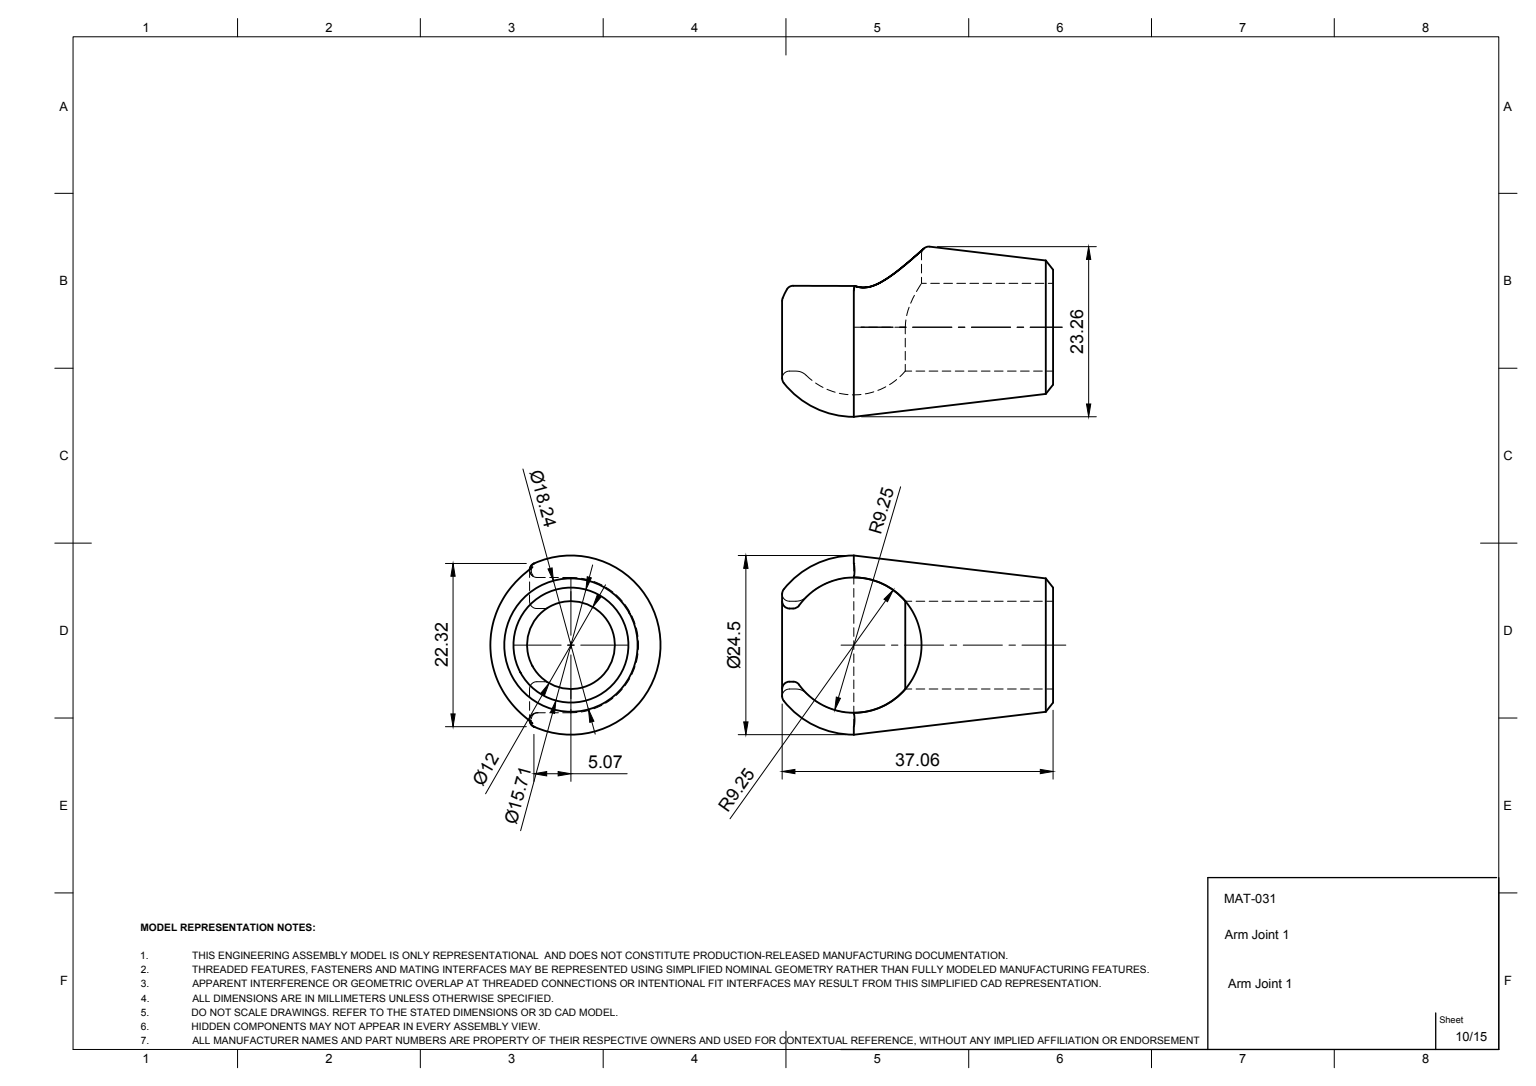
ISO-10303-21;
HEADER;
/* Generated by software containing ST-Developer
 * from STEP Tools, Inc. (www.steptools.com) 
 */

FILE_DESCRIPTION(
/* description */ ('STEP AP214'),
/* implementation_level */ '2;1');

FILE_NAME(
/* name */ 'Arm Joint 1.step',
/* time_stamp */ '2026-11-14T06:58:01-08:00',
/* author */ (''),
/* organization */ (''),
/* preprocessor_version */ 'ST-DEVELOPER v20.2',
/* originating_system */ 'Autodesk Translation Framework v15.17.0.0',
/* authorisation */ '');

FILE_SCHEMA (('AUTOMOTIVE_DESIGN { 1 0 10303 214 3 1 1 }'));
ENDSEC;

DATA;
#10=MECHANICAL_DESIGN_GEOMETRIC_PRESENTATION_REPRESENTATION('',(#1153),#38635);
#67=ELLIPSE('',#18082,0.093043907355238,0.0660721764139862);
#79=SPHERICAL_SURFACE('',#18062,1.);
#80=SPHERICAL_SURFACE('',#18074,9.25);
#81=SPHERICAL_SURFACE('',#18083,12.25);
#82=SPHERICAL_SURFACE('',#18107,1.);
#83=SPHERICAL_SURFACE('',#18111,1.);
#84=SPHERICAL_SURFACE('',#18115,1.);
#85=SPHERICAL_SURFACE('',#18118,1.);
#86=SPHERICAL_SURFACE('',#18123,1.);
#126=(
BOUNDED_SURFACE()
B_SPLINE_SURFACE(3,2,((#31255,#31256,#31257),(#31258,#31259,#31260),(#31261,
#31262,#31263),(#31264,#31265,#31266),(#31267,#31268,#31269),(#31270,#31271,
#31272),(#31273,#31274,#31275),(#31276,#31277,#31278),(#31279,#31280,#31281),
(#31282,#31283,#31284),(#31285,#31286,#31287),(#31288,#31289,#31290),(#31291,
#31292,#31293),(#31294,#31295,#31296),(#31297,#31298,#31299),(#31300,#31301,
#31302),(#31303,#31304,#31305),(#31306,#31307,#31308),(#31309,#31310,#31311),
(#31312,#31313,#31314),(#31315,#31316,#31317),(#31318,#31319,#31320),(#31321,
#31322,#31323),(#31324,#31325,#31326)),.UNSPECIFIED.,.F.,.F.,.F.)
B_SPLINE_SURFACE_WITH_KNOTS((4,2,2,2,2,2,2,2,2,2,2,4),(3,3),(-4.33680868994202E-19,
0.00199566610229966,0.00299349915344949,0.00399133220459933,0.00598699830689899,
0.00698483135804882,0.00748374788362374,0.00773320614641119,0.00785793527780492,
0.00792029984350179,0.00795148212635022,0.00798266440919865),(-8.88988013967173,
1.),.UNSPECIFIED.)
GEOMETRIC_REPRESENTATION_ITEM()
RATIONAL_B_SPLINE_SURFACE(((1.03673130903543,0.997934094247711,1.),(1.03429323702968,
0.998071220506301,1.),(1.03166096458261,0.99821926932168,1.),(1.02743039620336,
0.998457212258636,1.),(1.0259730109093,0.99853918104062,1.),(1.02296180766651,
0.998708542336582,1.),(1.02140250811888,0.998796243156116,1.),(1.01667872310722,
0.999061926435161,1.),(1.0134397522586,0.999244098230379,1.),(1.00845036900139,
0.999524719744889,1.),(1.00676184803489,0.99961968845875,1.),(1.00420736775411,
0.999763361952692,1.),(1.00335516609469,0.999811292950975,1.),(1.00207805691192,
0.999883122332401,1.),(1.00165222462761,0.999907072727549,1.),(1.00101619611475,
0.999942845342188,1.),(1.000804914933,0.999954728583493,1.),(1.00049166224454,
0.99997234708248,1.),(1.00038777606523,0.999978190028486,1.),(1.00023475952815,
0.999986796248967,1.),(1.00018401486096,0.999989650318224,1.),(1.00008917562832,
0.999994984430222,1.),(1.00003836348216,0.999997842294746,1.),(1.00003093298314,
0.999998260213712,1.)))
REPRESENTATION_ITEM('')
SURFACE()
);
#127=(
BOUNDED_SURFACE()
B_SPLINE_SURFACE(3,2,((#31328,#31329,#31330),(#31331,#31332,#31333),(#31334,
#31335,#31336),(#31337,#31338,#31339),(#31340,#31341,#31342),(#31343,#31344,
#31345),(#31346,#31347,#31348),(#31349,#31350,#31351),(#31352,#31353,#31354),
(#31355,#31356,#31357),(#31358,#31359,#31360),(#31361,#31362,#31363),(#31364,
#31365,#31366),(#31367,#31368,#31369),(#31370,#31371,#31372),(#31373,#31374,
#31375)),.UNSPECIFIED.,.F.,.F.,.F.)
B_SPLINE_SURFACE_WITH_KNOTS((4,2,2,2,2,2,2,4),(3,3),(-1.37073647788269E-16,
3.79857431933033E-5,7.59714863867437E-5,0.000151942972773624,0.000303885945547386,
0.000607771891094909,0.00121554378218996,0.00243108756438005),(-0.000101005518536674,
1.),.UNSPECIFIED.)
GEOMETRIC_REPRESENTATION_ITEM()
RATIONAL_B_SPLINE_SURFACE(((1.00000004220253,0.999791088022201,1.),(1.00000004430103,
0.999780699959677,1.),(1.00000006201562,0.999693008760642,1.),(1.00000010657676,
0.999472421084997,1.),(1.00000013303073,0.999341468019306,1.),(1.00000021861,
0.998917831394663,1.),(1.00000028470715,0.998590635693005,1.),(1.00000049900653,
0.997529805625635,1.),(1.00000066545063,0.996705869955465,1.),(1.00000123037801,
0.993909352546599,1.),(1.00000169504325,0.99160915523887,1.),(1.00000335151631,
0.983409241593269,1.),(1.00000480674396,0.976205537946754,1.),(1.00001025390194,
0.949240882635747,1.),(1.00001533088998,0.924108651696566,1.),(1.00002191434951,
0.891519048541741,1.)))
REPRESENTATION_ITEM('')
SURFACE()
);
#128=(
BOUNDED_SURFACE()
B_SPLINE_SURFACE(3,2,((#31377,#31378,#31379),(#31380,#31381,#31382),(#31383,
#31384,#31385),(#31386,#31387,#31388)),.UNSPECIFIED.,.F.,.F.,.F.)
B_SPLINE_SURFACE_WITH_KNOTS((4,4),(3,3),(-1.3918214625889E-5,0.00121512868205196),
(0.,1.00001391821463),.UNSPECIFIED.)
GEOMETRIC_REPRESENTATION_ITEM()
RATIONAL_B_SPLINE_SURFACE(((0.999999999999999,0.891779221283223,1.00000301248005),
(1.,0.884413245314419,1.00000321752252),(1.,0.87579683831728,1.00000345737252),
(1.,0.866200683852581,1.0000037244952)))
REPRESENTATION_ITEM('')
SURFACE()
);
#129=(
BOUNDED_SURFACE()
B_SPLINE_SURFACE(3,2,((#31400,#31401,#31402),(#31403,#31404,#31405),(#31406,
#31407,#31408),(#31409,#31410,#31411),(#31412,#31413,#31414),(#31415,#31416,
#31417),(#31418,#31419,#31420),(#31421,#31422,#31423),(#31424,#31425,#31426),
(#31427,#31428,#31429),(#31430,#31431,#31432),(#31433,#31434,#31435),(#31436,
#31437,#31438),(#31439,#31440,#31441)),.UNSPECIFIED.,.F.,.F.,.F.)
B_SPLINE_SURFACE_WITH_KNOTS((4,2,2,2,2,2,4),(3,3),(0.033103384374427,0.0355583288461946,
0.0367823574217915,0.0380063859973883,0.0392304145729851,0.0404544431485819,
0.0429025002997755),(0.,1.00000688732057),.UNSPECIFIED.)
GEOMETRIC_REPRESENTATION_ITEM()
RATIONAL_B_SPLINE_SURFACE(((1.,0.211850238456311,1.00001085648014),(1.,
0.211789774891773,1.000010857313),(1.,0.211720587176297,1.00001085826604),
(1.,0.21160403471626,1.0000108598715),(1.,0.211562868788471,1.00001086043855),
(1.,0.211477187752812,1.00001086161878),(1.,0.211433005503744,1.00001086222737),
(1.,0.211342033825223,1.00001086348047),(1.,0.211295244231205,1.00001086412498),
(1.,0.211199020809361,1.00001086545043),(1.,0.211149240972151,1.00001086613613),
(1.,0.21099910955097,1.00001086820413),(1.,0.210897693883658,1.0000108696011),
(1.,0.21079496787879,1.00001087101611)))
REPRESENTATION_ITEM('')
SURFACE()
);
#130=(
BOUNDED_SURFACE()
B_SPLINE_SURFACE(3,2,((#31518,#31519,#31520),(#31521,#31522,#31523),(#31524,
#31525,#31526),(#31527,#31528,#31529),(#31530,#31531,#31532),(#31533,#31534,
#31535),(#31536,#31537,#31538),(#31539,#31540,#31541),(#31542,#31543,#31544),
(#31545,#31546,#31547),(#31548,#31549,#31550),(#31551,#31552,#31553),(#31554,
#31555,#31556),(#31557,#31558,#31559),(#31560,#31561,#31562),(#31563,#31564,
#31565),(#31566,#31567,#31568),(#31569,#31570,#31571),(#31572,#31573,#31574),
(#31575,#31576,#31577),(#31578,#31579,#31580),(#31581,#31582,#31583),(#31584,
#31585,#31586),(#31587,#31588,#31589),(#31590,#31591,#31592),(#31593,#31594,
#31595),(#31596,#31597,#31598),(#31599,#31600,#31601),(#31602,#31603,#31604),
(#31605,#31606,#31607),(#31608,#31609,#31610),(#31611,#31612,#31613),(#31614,
#31615,#31616),(#31617,#31618,#31619),(#31620,#31621,#31622),(#31623,#31624,
#31625),(#31626,#31627,#31628),(#31629,#31630,#31631),(#31632,#31633,#31634),
(#31635,#31636,#31637),(#31638,#31639,#31640),(#31641,#31642,#31643),(#31644,
#31645,#31646),(#31647,#31648,#31649),(#31650,#31651,#31652),(#31653,#31654,
#31655),(#31656,#31657,#31658),(#31659,#31660,#31661),(#31662,#31663,#31664),
(#31665,#31666,#31667),(#31668,#31669,#31670),(#31671,#31672,#31673),(#31674,
#31675,#31676),(#31677,#31678,#31679),(#31680,#31681,#31682),(#31683,#31684,
#31685),(#31686,#31687,#31688),(#31689,#31690,#31691),(#31692,#31693,#31694),
(#31695,#31696,#31697),(#31698,#31699,#31700),(#31701,#31702,#31703),(#31704,
#31705,#31706),(#31707,#31708,#31709),(#31710,#31711,#31712),(#31713,#31714,
#31715),(#31716,#31717,#31718),(#31719,#31720,#31721),(#31722,#31723,#31724),
(#31725,#31726,#31727),(#31728,#31729,#31730),(#31731,#31732,#31733),(#31734,
#31735,#31736),(#31737,#31738,#31739),(#31740,#31741,#31742),(#31743,#31744,
#31745)),.UNSPECIFIED.,.F.,.F.,.F.)
B_SPLINE_SURFACE_WITH_KNOTS((4,2,2,2,2,2,2,2,2,2,2,2,2,2,2,2,2,2,2,2,2,
2,2,2,2,2,2,2,2,2,2,2,2,2,2,2,2,4),(3,3),(0.0155469420440516,0.0160999385621218,
0.016652935080192,0.0172059315982622,0.0177589281163324,0.0183119246344026,
0.0188649211524727,0.0194179176705429,0.0199709141886131,0.0210769072247535,
0.0221829002608939,0.0232888932970342,0.0243948863331746,0.025500879369315,
0.0266068724054554,0.0288188584777361,0.0299248515138765,0.0310308445500169,
0.0321368375861573,0.0332428306222976,0.034348823658438,0.0354548166945784,
0.0376668027668591,0.0398787888391399,0.0409847818752803,0.0420907749114206,
0.043196767947561,0.0443027609837014,0.0454087540198418,0.0465147470559821,
0.0470677435740523,0.0476207400921225,0.0481737366101927,0.0487267331282629,
0.0492797296463331,0.0498327261644033,0.0503857226824734,0.0509387192005436),
(0.,1.),.UNSPECIFIED.)
GEOMETRIC_REPRESENTATION_ITEM()
RATIONAL_B_SPLINE_SURFACE(((1.,0.229526735048257,1.),(1.,0.224133558219702,
1.),(1.,0.219259724176961,1.),(1.,0.211064181475465,1.),(1.,0.207811801710184,
1.),(1.,0.203341888285831,1.),(1.,0.202127973482812,1.),(1.,0.201960202180378,
1.),(1.,0.203032258888432,1.),(1.,0.207289559269388,1.),(1.,0.210454353335156,
1.),(1.,0.218450587215706,1.),(1.,0.223279069424003,1.),(1.,0.234195834429115,
1.),(1.,0.240233471751073,1.),(1.,0.252998923243242,1.),(1.,0.259742761586636,
1.),(1.,0.28067947683831,1.),(1.,0.295554256169214,1.),(1.,0.326016231928046,
1.),(1.,0.341634062441765,1.),(1.,0.372564100762139,1.),(1.,0.387951242324607,
1.),(1.,0.418305222299702,1.),(1.,0.433275214730199,1.),(1.,0.46261806682354,
1.),(1.,0.476992506609391,1.),(1.,0.504978264480088,1.),(1.,0.518645722843901,
1.),(1.,0.557478084599559,1.),(1.,0.580701256089758,1.),(1.,0.610367709572221,
1.),(1.,0.619422302565764,1.),(1.,0.635083430287347,1.),(1.,0.64175221457835,
1.),(1.,0.65261413861016,1.),(1.,0.656808227795975,1.),(1.,0.662484548907152,
1.),(1.,0.663913234852522,1.),(1.,0.663922009369197,1.),(1.,0.66252245378572,
1.),(1.,0.656942975295251,1.),(1.,0.652711192029527,1.),(1.,0.636300872830255,
1.),(1.,0.620465569188766,1.),(1.,0.580610974593483,1.),(1.,0.557339096866905,
1.),(1.,0.518721884857682,1.),(1.,0.505222106533921,1.),(1.,0.477115614134931,
1.),(1.,0.462576289466857,1.),(1.,0.433080321145928,1.),(1.,0.418066573341961,
1.),(1.,0.387696762864547,1.),(1.,0.372337606905373,1.),(1.,0.341539686788467,
1.),(1.,0.326093173961657,1.),(1.,0.295606321651459,1.),(1.,0.280553638483726,
1.),(1.,0.25953297193159,1.),(1.,0.252774217996814,1.),(1.,0.240006731870622,
1.),(1.,0.233989040402757,1.),(1.,0.223104380065769,1.),(1.,0.218299068913211,
1.),(1.,0.210355245717533,1.),(1.,0.207219723680965,1.),(1.,0.203010941824996,
1.),(1.,0.201948260378419,1.),(1.,0.202143131871967,1.),(1.,0.203375531025685,
1.),(1.,0.207855714464755,1.),(1.,0.211099729925129,1.),(1.,0.219230361697907,
1.),(1.,0.224140752438636,1.),(1.,0.229539201120578,1.)))
REPRESENTATION_ITEM('')
SURFACE()
);
#131=(
BOUNDED_SURFACE()
B_SPLINE_SURFACE(3,2,((#31822,#31823,#31824),(#31825,#31826,#31827),(#31828,
#31829,#31830),(#31831,#31832,#31833),(#31834,#31835,#31836),(#31837,#31838,
#31839),(#31840,#31841,#31842),(#31843,#31844,#31845),(#31846,#31847,#31848),
(#31849,#31850,#31851),(#31852,#31853,#31854),(#31855,#31856,#31857),(#31858,
#31859,#31860),(#31861,#31862,#31863)),.UNSPECIFIED.,.F.,.F.,.F.)
B_SPLINE_SURFACE_WITH_KNOTS((4,2,2,2,2,2,4),(3,3),(0.0331033843745195,0.0355583288461946,
0.0367823574217914,0.0380063859973882,0.039230414572985,0.0404544431485818,
0.0429025002997754),(-6.88732048148063E-6,1.),.UNSPECIFIED.)
GEOMETRIC_REPRESENTATION_ITEM()
RATIONAL_B_SPLINE_SURFACE(((1.00001085647999,0.211850238456374,0.999999999999999),
(1.00001085731285,0.211789774892188,1.),(1.00001085826589,0.211720587175911,
1.),(1.00001085987136,0.211604034716559,1.),(1.0000108604384,0.211562868788407,
1.),(1.00001086161863,0.211477187753023,1.),(1.00001086222722,0.211433005503953,
1.),(1.00001086348033,0.21134203382516,1.),(1.00001086412484,0.211295244231278,
1.),(1.00001086545028,0.211199020809434,1.),(1.00001086613598,0.211149240972224,
1.),(1.00001086820399,0.210999109551043,1.),(1.00001086960095,0.21089769388373,
1.),(1.00001087101596,0.210794967878863,1.)))
REPRESENTATION_ITEM('')
SURFACE()
);
#132=(
BOUNDED_SURFACE()
B_SPLINE_SURFACE(3,2,((#31872,#31873,#31874),(#31875,#31876,#31877),(#31878,
#31879,#31880),(#31881,#31882,#31883)),.UNSPECIFIED.,.F.,.F.,.F.)
B_SPLINE_SURFACE_WITH_KNOTS((4,4),(3,3),(-1.39182146545714E-5,0.00121512868208074),
(0.,1.00001391821465),.UNSPECIFIED.)
GEOMETRIC_REPRESENTATION_ITEM()
RATIONAL_B_SPLINE_SURFACE(((1.,0.866200683851906,1.00000372449521),(1.,
0.875796838317096,1.00000345737253),(1.,0.884413245314652,1.00000321752253),
(1.,0.891779221283738,1.00000301248006)))
REPRESENTATION_ITEM('')
SURFACE()
);
#133=(
BOUNDED_SURFACE()
B_SPLINE_SURFACE(3,2,((#31885,#31886,#31887),(#31888,#31889,#31890),(#31891,
#31892,#31893),(#31894,#31895,#31896),(#31897,#31898,#31899),(#31900,#31901,
#31902),(#31903,#31904,#31905),(#31906,#31907,#31908),(#31909,#31910,#31911),
(#31912,#31913,#31914),(#31915,#31916,#31917),(#31918,#31919,#31920),(#31921,
#31922,#31923),(#31924,#31925,#31926)),.UNSPECIFIED.,.F.,.F.,.F.)
B_SPLINE_SURFACE_WITH_KNOTS((4,2,2,2,2,2,4),(3,3),(-0.000142750203022182,
0.00120936219001056,0.00181404328501584,0.00211638383251848,0.0022675541062698,
0.00234313924314546,0.0025614745830495),(-0.00757884796103774,1.),
 .UNSPECIFIED.)
GEOMETRIC_REPRESENTATION_ITEM()
RATIONAL_B_SPLINE_SURFACE(((1.00183804612443,0.878738422126962,1.),(1.00124990939078,
0.917539618342774,1.),(1.00080710421406,0.946752843030485,1.),(1.00036309214798,
0.976045689935564,1.),(1.00025309503348,0.983302539200046,1.),(1.00012791013031,
0.991561373775666,1.),(1.00009280627034,0.993877283802622,1.),(1.00005012171262,
0.996693315865673,1.),(1.00003753469437,0.997523720322227,1.),(1.00002137280872,
0.998589969819041,1.),(1.00001641874054,0.998916804993093,1.),(0.999999713951067,
1.00001887153131,1.),(0.999989596975289,1.00068631965997,1.),(1.00005723328726,
0.996224143329086,0.999999999999999)))
REPRESENTATION_ITEM('')
SURFACE()
);
#134=(
BOUNDED_SURFACE()
B_SPLINE_SURFACE(3,2,((#31928,#31929,#31930),(#31931,#31932,#31933),(#31934,
#31935,#31936),(#31937,#31938,#31939),(#31940,#31941,#31942),(#31943,#31944,
#31945),(#31946,#31947,#31948),(#31949,#31950,#31951),(#31952,#31953,#31954),
(#31955,#31956,#31957),(#31958,#31959,#31960),(#31961,#31962,#31963),(#31964,
#31965,#31966),(#31967,#31968,#31969),(#31970,#31971,#31972),(#31973,#31974,
#31975),(#31976,#31977,#31978),(#31979,#31980,#31981),(#31982,#31983,#31984),
(#31985,#31986,#31987),(#31988,#31989,#31990),(#31991,#31992,#31993),(#31994,
#31995,#31996),(#31997,#31998,#31999)),.UNSPECIFIED.,.F.,.F.,.F.)
B_SPLINE_SURFACE_WITH_KNOTS((4,2,2,2,2,2,2,2,2,2,2,4),(3,3),(0.,0.00199566610230272,
0.00299349915345408,0.00399133220460544,0.00598699830690816,0.00698483135805952,
0.0074837478836352,0.00773320614642304,0.00785793527781696,0.00792029984351392,
0.0079514821263624,0.00798266440921088),(0.,9.4347309660509),
 .UNSPECIFIED.)
GEOMETRIC_REPRESENTATION_ITEM()
RATIONAL_B_SPLINE_SURFACE(((1.,0.998029170758512,1.03324682886395),(1.,
0.99815998623251,1.03104004220522),(1.,0.998301221588568,1.02865747774274),
(1.,0.998528213985216,1.02482823814861),(1.,0.99860641042422,1.0235091062976),
(1.,0.998767977423409,1.0207835579553),(1.,0.998851642101808,1.01937217984798),
(1.,0.999105098182627,1.01509651214116),(1.,0.999278886120722,1.01216480313518),
(1.,0.999546592953898,1.00764873290395),(1.,0.999637191045363,1.00612039184888),
(1.,0.999774252439753,1.00380823987384),(1.,0.999819977571642,1.00303688150212),
(1.,0.999888501242266,1.00188092404907),(1.,0.999911349399373,1.00149548793254),
(1.,0.99994547569713,1.00091979565164),(1.,0.999956812051398,1.00072855745488),
(1.,0.999973619716972,1.0004450211803),(1.,0.999979193760625,1.00035099006309),
(1.,0.999987403908142,1.0002124892921),(1.,0.999990126628257,1.00016655846877),
(1.,0.999995215255311,1.00008071606839),(1.,0.999997941596032,1.00003472416737),
(1.,0.999998340281648,1.00002799855556)))
REPRESENTATION_ITEM('')
SURFACE()
);
#145=TOROIDAL_SURFACE('',#18066,7.,0.999999999999999);
#146=TOROIDAL_SURFACE('',#18072,8.,2.);
#147=TOROIDAL_SURFACE('',#18113,9.51643315533714,1.);
#148=TOROIDAL_SURFACE('',#18120,9.51643315533713,1.);
#875=FACE_BOUND('',#2837,.T.);
#965=B_SPLINE_CURVE_WITH_KNOTS('',3,(#30002,#30003,#30004,#30005,#30006,
#30007,#30008,#30009,#30010,#30011),.UNSPECIFIED.,.F.,.F.,(4,3,3,4),(9.57246758340288E-17,
0.000355403916957923,0.000707000583199714,0.00104888238406079),
 .UNSPECIFIED.);
#966=B_SPLINE_CURVE_WITH_KNOTS('',3,(#30015,#30016,#30017,#30018,#30019,
#30020,#30021,#30022,#30023,#30024),.UNSPECIFIED.,.F.,.F.,(4,3,3,4),(0.,
0.00035058235323811,0.000705441803886655,0.0010488823840608),
 .UNSPECIFIED.);
#967=B_SPLINE_CURVE_WITH_KNOTS('',3,(#30030,#30031,#30032,#30033,#30034,
#30035,#30036,#30037,#30038,#30039,#30040,#30041,#30042,#30043,#30044,#30045,
#30046,#30047,#30048,#30049,#30050,#30051,#30052,#30053,#30054,#30055,#30056,
#30057,#30058,#30059,#30060,#30061,#30062,#30063,#30064,#30065,#30066,#30067,
#30068,#30069,#30070,#30071,#30072,#30073,#30074,#30075,#30076,#30077,#30078,
#30079,#30080,#30081,#30082,#30083,#30084,#30085,#30086,#30087,#30088,#30089,
#30090,#30091,#30092,#30093,#30094,#30095,#30096),.UNSPECIFIED.,.F.,.F.,
(4,3,3,3,3,3,3,3,3,3,3,3,3,3,3,3,3,3,3,3,3,3,4),(1.12014731928769E-16,2.44686880794631E-5,
5.01962031411245E-5,6.46659802217382E-5,9.34320062910693E-5,0.000117250238179507,
0.0001221980323604,0.000160663500114897,0.000207281263733168,0.000216514808073292,
0.000286414601198953,0.000321327000229682,0.000388105160880686,0.000522741781205867,
0.000642654000459244,0.000713976475490795,0.000947916545100924,0.00121389085366499,
0.00128530800091837,0.0013411477040794,0.00178543654748138,0.00228581177424824,
0.00257061600183662),.UNSPECIFIED.);
#968=B_SPLINE_CURVE_WITH_KNOTS('',3,(#30097,#30098,#30099,#30100,#30101,
#30102,#30103,#30104,#30105,#30106,#30107,#30108,#30109,#30110,#30111,#30112,
#30113,#30114,#30115,#30116,#30117,#30118,#30119,#30120,#30121,#30122,#30123,
#30124,#30125,#30126,#30127,#30128,#30129,#30130,#30131,#30132,#30133,#30134,
#30135,#30136,#30137,#30138,#30139,#30140,#30141,#30142,#30143,#30144,#30145,
#30146,#30147,#30148,#30149,#30150,#30151,#30152,#30153,#30154,#30155,#30156,
#30157),.UNSPECIFIED.,.F.,.F.,(4,3,3,3,3,3,3,3,3,3,3,3,3,3,3,3,3,3,3,3,
4),(0.,0.00046515412756322,0.000882411108678421,0.0012173266037486,0.00127005672264322,
0.00158659639906562,0.00183772251820228,0.00190508508396483,0.00203713318246821,
0.00215739978931402,0.00222259926462564,0.00227522662628161,0.00232413118357583,
0.00232785398793758,0.00236109891842404,0.00238135635495604,0.00242717801579792,
0.00245270320014808,0.0024836859974019,0.00251622256417103,0.00254011344528644),
 .UNSPECIFIED.);
#969=B_SPLINE_CURVE_WITH_KNOTS('',3,(#30160,#30161,#30162,#30163,#30164,
#30165,#30166,#30167,#30168,#30169,#30170,#30171,#30172,#30173,#30174,#30175,
#30176,#30177,#30178,#30179,#30180,#30181,#30182,#30183,#30184,#30185,#30186,
#30187,#30188,#30189,#30190,#30191,#30192,#30193,#30194,#30195,#30196,#30197,
#30198,#30199,#30200,#30201,#30202,#30203,#30204,#30205,#30206,#30207,#30208,
#30209,#30210,#30211,#30212,#30213,#30214,#30215,#30216,#30217,#30218,#30219,
#30220,#30221,#30222,#30223,#30224,#30225,#30226),.UNSPECIFIED.,.F.,.F.,
(4,3,3,3,3,3,3,3,3,3,3,3,3,3,3,3,3,3,3,3,3,3,4),(6.34356547860961E-12,2.91015092365536E-5,
2.91145195680595E-5,5.82134784524454E-5,5.8229039136119E-5,0.000116442640098838,
0.000116458078272238,0.000232900963425353,0.000232916156544486,0.000465817610066878,
0.000465832313088972,0.000931650903358755,0.000931664626177945,0.0018633174899382,
0.00186332925235589,0.00372665066309962,0.00372665850471178,0.00465831724968086,
0.00465832313088973,0.0055899838362617,0.00558998775706768,0.00723192026679969,
0.00745331700942357),.UNSPECIFIED.);
#970=B_SPLINE_CURVE_WITH_KNOTS('',3,(#30228,#30229,#30230,#30231,#30232,
#30233,#30234,#30235,#30236,#30237,#30238,#30239,#30240,#30241,#30242,#30243,
#30244,#30245,#30246,#30247,#30248,#30249,#30250,#30251,#30252,#30253,#30254,
#30255,#30256,#30257,#30258,#30259,#30260,#30261,#30262,#30263,#30264,#30265,
#30266,#30267,#30268,#30269,#30270,#30271,#30272,#30273,#30274,#30275,#30276,
#30277,#30278,#30279,#30280,#30281,#30282,#30283,#30284,#30285,#30286,#30287,
#30288,#30289,#30290,#30291,#30292,#30293,#30294),.UNSPECIFIED.,.F.,.F.,
(4,3,3,3,3,3,3,3,3,3,3,3,3,3,3,3,3,3,3,3,3,3,4),(4.33816373096554E-18,0.00158697662988317,
0.00180096318079261,0.00180096697037075,0.00270144477118891,0.0027014504555561,
0.00360192636158522,0.00360193394074181,0.00540288954237782,0.00540290091111227,
0.00630337113277412,0.00630338439629625,0.00675361192797227,0.00675362613889033,
0.00697873232557134,0.0069787470101831,0.00709129252437088,0.00709130744503989,
0.00714757262377064,0.00714758767823208,0.00717571267347053,0.00717572524835171,
0.00719063527707478),.UNSPECIFIED.);
#971=B_SPLINE_CURVE_WITH_KNOTS('',3,(#30298,#30299,#30300,#30301),
 .UNSPECIFIED.,.F.,.F.,(4,4),(0.00719063527707478,0.00720385271268794),
 .UNSPECIFIED.);
#972=B_SPLINE_CURVE_WITH_KNOTS('',3,(#30310,#30311,#30312,#30313,#30314,
#30315,#30316,#30317,#30318,#30319,#30320,#30321,#30322,#30323,#30324,#30325,
#30326,#30327,#30328,#30329,#30330,#30331,#30332,#30333,#30334,#30335,#30336,
#30337,#30338,#30339,#30340,#30341,#30342,#30343,#30344,#30345,#30346,#30347,
#30348,#30349,#30350,#30351,#30352,#30353,#30354,#30355,#30356,#30357,#30358,
#30359,#30360,#30361,#30362,#30363,#30364,#30365,#30366,#30367,#30368,#30369,
#30370,#30371,#30372,#30373,#30374,#30375,#30376,#30377,#30378,#30379,#30380,
#30381,#30382,#30383,#30384,#30385,#30386,#30387,#30388,#30389,#30390,#30391,
#30392,#30393,#30394,#30395,#30396,#30397,#30398,#30399,#30400,#30401,#30402,
#30403,#30404,#30405,#30406,#30407,#30408,#30409,#30410,#30411,#30412,#30413,
#30414,#30415,#30416,#30417,#30418,#30419,#30420,#30421,#30422,#30423,#30424,
#30425,#30426,#30427,#30428,#30429,#30430,#30431,#30432,#30433,#30434,#30435,
#30436),.UNSPECIFIED.,.F.,.F.,(4,3,3,3,3,3,3,3,3,3,3,3,3,3,3,3,3,3,3,3,
3,3,3,3,3,3,3,3,3,3,3,3,3,3,3,3,3,3,3,3,3,3,4),(0.0187104358930852,0.0198797262251292,
0.0199481217388706,0.0207658399883224,0.0210490165571731,0.021186081177019,
0.0227741969642194,0.0233875972212611,0.0236455138385063,0.0244983758541658,
0.024556887553305,0.0254911534667947,0.025726177885349,0.0260776320456601,
0.026895468217393,0.0272825913183847,0.0278847304061735,0.028064758549437,
0.0284807962042684,0.0294503982294847,0.0296719241460166,0.0304033392135249,
0.0308553085637769,0.0315726295455689,0.0320297867900004,0.032682244583055,
0.0327419198776128,0.0331939007038932,0.0337336131064912,0.0337714568809753,
0.0339112102096568,0.034345218787789,0.0349152553128406,0.0350805005417007,
0.0354825389403645,0.0356651457077227,0.0359067035564612,0.0360469991704175,
0.0362497908737447,0.0366116523092686,0.0370487581095643,0.0371780544079827,
0.0374190812057887),.UNSPECIFIED.);
#973=B_SPLINE_CURVE_WITH_KNOTS('',3,(#30438,#30439,#30440,#30441,#30442,
#30443),.UNSPECIFIED.,.F.,.F.,(4,2,4),(-0.00187765892693451,-0.00093532678058844,
-6.51826565449196E-7),.UNSPECIFIED.);
#974=B_SPLINE_CURVE_WITH_KNOTS('',3,(#30451,#30452,#30453,#30454,#30455,
#30456,#30457,#30458,#30459,#30460,#30461,#30462,#30463,#30464,#30465,#30466,
#30467,#30468,#30469,#30470,#30471,#30472,#30473,#30474,#30475,#30476,#30477,
#30478,#30479,#30480,#30481,#30482,#30483,#30484,#30485,#30486,#30487,#30488,
#30489,#30490,#30491,#30492,#30493,#30494,#30495,#30496,#30497,#30498,#30499,
#30500,#30501,#30502,#30503,#30504,#30505,#30506,#30507,#30508,#30509,#30510,
#30511,#30512,#30513,#30514,#30515,#30516,#30517,#30518,#30519,#30520,#30521,
#30522,#30523,#30524,#30525,#30526,#30527,#30528,#30529,#30530,#30531,#30532,
#30533,#30534,#30535,#30536,#30537,#30538,#30539,#30540,#30541,#30542,#30543,
#30544,#30545,#30546,#30547,#30548,#30549,#30550,#30551,#30552,#30553,#30554,
#30555,#30556,#30557,#30558,#30559,#30560,#30561,#30562,#30563,#30564,#30565,
#30566,#30567,#30568,#30569,#30570,#30571,#30572,#30573,#30574,#30575,#30576,
#30577,#30578,#30579,#30580,#30581,#30582,#30583,#30584,#30585,#30586,#30587,
#30588,#30589,#30590,#30591,#30592),.UNSPECIFIED.,.F.,.F.,(4,3,3,3,3,3,
3,3,3,3,3,3,3,3,3,3,3,3,3,3,3,3,3,3,3,3,3,3,3,3,3,3,3,3,3,3,3,3,3,3,3,3,
3,3,3,3,3,4),(1.4149286155699E-6,0.00024128475743038,0.000632178371154065,
0.000806980085871294,0.00117072873889494,0.00137185559650634,0.00175538564403461,
0.00193588458492275,0.00229633258208871,0.00234004254917429,0.00250284011366328,
0.00292469945431397,0.00307277910263342,0.00345879313729314,0.00350935635945365,
0.00364629450818616,0.00422381295371362,0.004678670169733,0.00533094003789352,
0.00538807166103802,0.00606788887869631,0.00656252330787629,0.00701729779029169,
0.00774578828639105,0.0088092112391015,0.0089367826515657,0.00935592541085039,
0.0101349902304355,0.0105252392211297,0.0112073453952734,0.0113400647033204,
0.0116945530314091,0.0125954135092807,0.0134677368138639,0.0137717393674888,
0.0140331806519678,0.0146914487977971,0.0149985613295519,0.0152024944622471,
0.0162308220365952,0.0163718082725265,0.016968388316562,0.0174681862798869,
0.0175411220828058,0.0180728185856757,0.0186062516405492,0.0187085025636743,
0.0187104358930852),.UNSPECIFIED.);
#975=B_SPLINE_CURVE_WITH_KNOTS('',3,(#30596,#30597,#30598,#30599,#30600,
#30601,#30602,#30603,#30604,#30605,#30606,#30607,#30608,#30609),
 .UNSPECIFIED.,.F.,.F.,(4,2,2,2,2,2,4),(2.60208521396521E-18,0.00261973771586097,
0.00392960657379145,0.00523947543172193,0.00654934428965241,0.00785921314758289,
0.0104789508634439),.UNSPECIFIED.);
#976=B_SPLINE_CURVE_WITH_KNOTS('',3,(#30611,#30612,#30613,#30614,#30615,
#30616,#30617,#30618,#30619,#30620,#30621,#30622,#30623,#30624),
 .UNSPECIFIED.,.F.,.F.,(4,2,2,2,2,2,4),(6.14713909703637E-8,0.00263335930455818,
0.00395003895683728,0.00526671860911637,0.00658339826139546,0.00790007791367455,
0.0105334372182327),.UNSPECIFIED.);
#977=B_SPLINE_CURVE_WITH_KNOTS('',3,(#30630,#30631,#30632,#30633,#30634,
#30635,#30636,#30637,#30638,#30639),.UNSPECIFIED.,.F.,.F.,(4,2,2,2,4),(0.,
0.23587669570582,0.471753391411641,0.705378949636768,0.939004507861895),
 .UNSPECIFIED.);
#978=B_SPLINE_CURVE_WITH_KNOTS('',3,(#30644,#30645,#30646,#30647,#30648,
#30649,#30650,#30651,#30652,#30653),.UNSPECIFIED.,.F.,.F.,(4,2,2,2,4),(0.939004507861895,
1.17263006608702,1.40625562431215,1.64213232001797,1.87800901572379),
 .UNSPECIFIED.);
#979=B_SPLINE_CURVE_WITH_KNOTS('',3,(#30662,#30663,#30664,#30665,#30666,
#30667,#30668,#30669,#30670,#30671,#30672,#30673,#30674,#30675,#30676,#30677,
#30678,#30679,#30680,#30681,#30682,#30683,#30684,#30685,#30686,#30687,#30688,
#30689,#30690,#30691,#30692,#30693,#30694,#30695,#30696,#30697,#30698,#30699,
#30700,#30701,#30702,#30703,#30704,#30705,#30706,#30707,#30708,#30709,#30710,
#30711,#30712,#30713,#30714,#30715,#30716,#30717,#30718,#30719,#30720,#30721,
#30722,#30723,#30724,#30725,#30726,#30727,#30728,#30729,#30730,#30731,#30732,
#30733,#30734,#30735,#30736,#30737,#30738,#30739,#30740),.UNSPECIFIED.,
 .F.,.F.,(4,3,3,3,3,3,3,3,3,3,3,3,3,3,3,3,3,3,3,3,3,3,3,3,3,3,4),(1.48114181800469E-12,
1.62713353573857E-5,2.85253456785481E-5,2.91748611457617E-5,3.0602416023118E-5,
5.19981524978168E-5,5.83497222915234E-5,6.03636063786387E-5,0.000116699444583057,
0.000119109456676927,0.000233398889166133,0.000236199927572212,0.000466797778332297,
0.000469925964041112,0.000933595556664625,0.000936857543433071,0.00186719111332928,
0.00187024522129993,0.00362565651164336,0.00373438222665858,0.00373660042866314,
0.00466797778332323,0.00466967995109927,0.00560157333998787,0.00560272875185939,
0.00726089770434782,0.00746876445331715),.UNSPECIFIED.);
#980=B_SPLINE_CURVE_WITH_KNOTS('',3,(#30742,#30743,#30744,#30745,#30746,
#30747,#30748,#30749,#30750,#30751,#30752,#30753,#30754,#30755,#30756,#30757),
 .UNSPECIFIED.,.F.,.F.,(4,2,2,2,2,2,2,4),(0.,3.69926380493027E-5,7.39852760986054E-5,
0.000147970552197207,0.000295941104394409,0.000591882208788816,0.00118376441757763,
0.00236752883515526),.UNSPECIFIED.);
#981=B_SPLINE_CURVE_WITH_KNOTS('',3,(#30759,#30760,#30761,#30762,#30763,
#30764,#30765),.UNSPECIFIED.,.F.,.F.,(4,3,4),(0.,0.000624637568767089,0.00116946841139767),
 .UNSPECIFIED.);
#982=B_SPLINE_CURVE_WITH_KNOTS('',3,(#30769,#30770,#30771,#30772,#30773,
#30774,#30775,#30776,#30777,#30778,#30779,#30780,#30781,#30782),
 .UNSPECIFIED.,.F.,.F.,(4,2,2,2,2,2,4),(0.,0.00215799408414667,0.00323699112622001,
0.00431598816829334,0.00539498521036668,0.00647398225244002,0.00863197633658669),
 .UNSPECIFIED.);
#983=B_SPLINE_CURVE_WITH_KNOTS('',3,(#30784,#30785,#30786,#30787,#30788,
#30789,#30790,#30791,#30792,#30793,#30794,#30795,#30796,#30797,#30798,#30799,
#30800,#30801,#30802,#30803,#30804,#30805,#30806,#30807,#30808,#30809,#30810,
#30811,#30812,#30813,#30814,#30815,#30816,#30817,#30818,#30819,#30820,#30821,
#30822,#30823,#30824,#30825,#30826,#30827,#30828,#30829,#30830,#30831,#30832,
#30833,#30834,#30835,#30836,#30837,#30838,#30839,#30840,#30841,#30842,#30843,
#30844,#30845,#30846,#30847,#30848,#30849,#30850,#30851,#30852,#30853,#30854,
#30855,#30856,#30857,#30858,#30859,#30860,#30861,#30862,#30863,#30864,#30865,
#30866,#30867,#30868,#30869,#30870,#30871,#30872,#30873,#30874,#30875,#30876,
#30877,#30878,#30879,#30880,#30881,#30882,#30883,#30884,#30885,#30886,#30887,
#30888,#30889,#30890,#30891,#30892,#30893,#30894,#30895,#30896,#30897,#30898,
#30899,#30900,#30901,#30902,#30903,#30904,#30905,#30906,#30907,#30908,#30909,
#30910,#30911,#30912,#30913,#30914,#30915,#30916,#30917,#30918,#30919,#30920,
#30921,#30922,#30923,#30924,#30925,#30926,#30927,#30928,#30929,#30930,#30931,
#30932,#30933,#30934,#30935,#30936,#30937,#30938,#30939,#30940,#30941,#30942,
#30943,#30944,#30945,#30946,#30947,#30948,#30949,#30950,#30951,#30952,#30953,
#30954,#30955,#30956,#30957,#30958,#30959,#30960,#30961,#30962,#30963,#30964,
#30965,#30966,#30967,#30968,#30969,#30970,#30971,#30972,#30973,#30974,#30975,
#30976,#30977,#30978,#30979,#30980,#30981,#30982,#30983,#30984,#30985,#30986,
#30987,#30988,#30989,#30990,#30991,#30992,#30993,#30994,#30995,#30996,#30997,
#30998,#30999,#31000,#31001,#31002,#31003,#31004,#31005,#31006,#31007,#31008,
#31009,#31010,#31011,#31012,#31013,#31014,#31015,#31016,#31017,#31018,#31019,
#31020,#31021,#31022,#31023,#31024,#31025,#31026,#31027),.UNSPECIFIED.,
 .F.,.F.,(4,3,3,3,3,3,3,3,3,3,3,3,3,3,3,3,3,3,3,3,3,3,3,3,3,3,3,3,3,3,3,
3,3,3,3,3,3,3,3,3,3,3,3,3,3,3,3,3,3,3,3,3,3,3,3,3,3,3,3,3,3,3,3,3,3,3,3,
3,3,3,3,3,3,3,3,3,3,3,3,3,3,4),(6.64190588068549E-10,0.00015883717919967,
0.000661562575487372,0.000994806103415245,0.00116260554575537,0.00138085520112917,
0.00149220915512287,0.00166326601977262,0.00198961220683049,0.00216588071655761,
0.00267030663113129,0.00298441831024573,0.00317737089357229,0.00368692950170913,
0.00397922441366098,0.00458731308453751,0.00471140773606946,0.00497403051707622,
0.00573980998888102,0.00596883662049147,0.00676961605918934,0.00779952990691134,
0.00795844882732194,0.008643398393127,0.0088280406155012,0.00895325493073719,
0.00985354333845186,0.00994806103415243,0.010673080413176,0.0113658404477328,
0.011891944708529,0.0119376732409829,0.0126851783449462,0.013408573202733,
0.0139116067056583,0.0139272854478134,0.0144550918417944,0.0149150434308082,
0.0149220915512286,0.0159168976546438,0.0159173041609428,0.0165518344898443,
0.0169117037580591,0.0169188369330008,0.0176391579183572,0.0179065098614743,
0.0179228529559086,0.0189013159648895,0.0189308538029226,0.0195006539338095,
0.0198961220683048,0.0199428610575756,0.0209581619462027,0.0218857342751353,
0.0219816750595829,0.0226544548355501,0.0228805403785505,0.0230073178663708,
0.0237710581938644,0.0238753464819657,0.0240355283687645,0.0250012828336967,
0.0250653536857579,0.0258649586887962,0.0260955990941479,0.026789820669263,
0.0271245982346018,0.0277221457004299,0.0278545708956267,0.0281492510550362,
0.028658852638223,0.0288493769990419,0.0291659944242556,0.0296702290396597,
0.0298441831024571,0.0301723844621069,0.0305140708508808,0.0306728710844153,
0.0308389892058724,0.0311737826503289,0.031675697204179,0.0318337953069872),
 .UNSPECIFIED.);
#984=B_SPLINE_CURVE_WITH_KNOTS('',3,(#31029,#31030,#31031,#31032,#31033,
#31034,#31035,#31036,#31037,#31038,#31039,#31040,#31041,#31042),
 .UNSPECIFIED.,.F.,.F.,(4,2,2,2,2,2,4),(0.,0.00217004055772761,0.00325506083659142,
0.00434008111545523,0.00542510139431905,0.00651012167318285,0.00868016223091047),
 .UNSPECIFIED.);
#985=B_SPLINE_CURVE_WITH_KNOTS('',3,(#31046,#31047,#31048,#31049,#31050,
#31051,#31052),.UNSPECIFIED.,.F.,.F.,(4,3,4),(1.93947980722443E-18,0.000624637568797489,
0.00116946841139767),.UNSPECIFIED.);
#986=B_SPLINE_CURVE_WITH_KNOTS('',3,(#31054,#31055,#31056,#31057,#31058,
#31059,#31060,#31061,#31062,#31063,#31064,#31065,#31066,#31067,#31068,#31069,
#31070,#31071,#31072,#31073,#31074,#31075,#31076,#31077,#31078,#31079,#31080,
#31081,#31082,#31083,#31084,#31085,#31086,#31087,#31088,#31089,#31090,#31091,
#31092,#31093,#31094,#31095,#31096,#31097,#31098,#31099,#31100,#31101,#31102,
#31103,#31104,#31105,#31106,#31107,#31108,#31109,#31110,#31111,#31112,#31113,
#31114,#31115,#31116,#31117,#31118,#31119,#31120,#31121,#31122,#31123,#31124,
#31125,#31126,#31127,#31128,#31129,#31130,#31131,#31132,#31133,#31134,#31135,
#31136,#31137,#31138,#31139,#31140,#31141,#31142,#31143,#31144,#31145,#31146,
#31147,#31148,#31149,#31150,#31151,#31152,#31153,#31154,#31155,#31156),
 .UNSPECIFIED.,.F.,.F.,(4,3,3,3,3,3,3,3,3,3,3,3,3,3,3,3,3,3,3,3,3,3,3,3,
3,3,3,3,3,3,3,3,3,3,4),(0.,0.000848753575416885,0.00118770142037617,0.00118810169232347,
0.00178155213056426,0.00178416675818213,0.00193001480811129,0.00207847748565831,
0.00208223092752585,0.00215270882443182,0.00218982449381858,0.00222694016320533,
0.0022307594594149,0.00224549799789871,0.00225245718590873,0.00227681434394379,
0.00228899292296132,0.0022920375677157,0.00230117150197885,0.00230441261012628,
0.00231045041932553,0.00231219021632804,0.00231300574617296,0.00231379579071023,
0.00232604148103792,0.00233216432620176,0.00233369503749272,0.00233426905422683,
0.0023382871713656,0.00234060924917293,0.00234756608871229,0.00234843598721354,
0.00234927870138663,0.00236769555909942,0.00237540284075236),
 .UNSPECIFIED.);
#987=B_SPLINE_CURVE_WITH_KNOTS('',3,(#31157,#31158,#31159,#31160,#31161,
#31162,#31163,#31164,#31165,#31166,#31167,#31168,#31169,#31170,#31171,#31172,
#31173,#31174,#31175,#31176,#31177,#31178,#31179,#31180,#31181,#31182,#31183,
#31184,#31185,#31186,#31187,#31188,#31189,#31190,#31191,#31192,#31193,#31194,
#31195,#31196,#31197,#31198,#31199,#31200,#31201,#31202,#31203,#31204,#31205,
#31206,#31207,#31208,#31209,#31210,#31211,#31212,#31213,#31214,#31215,#31216,
#31217,#31218,#31219,#31220,#31221,#31222,#31223,#31224,#31225,#31226,#31227,
#31228,#31229,#31230,#31231,#31232,#31233,#31234,#31235),.UNSPECIFIED.,
 .F.,.F.,(4,3,3,3,3,3,3,3,3,3,3,3,3,3,3,3,3,3,3,3,3,3,3,3,3,3,4),(0.,0.00160045154295414,
0.00180108286976027,0.00180219806414393,0.00270165417736523,0.00270329709621589,
0.00360225513728841,0.00360439612828786,0.0052987050646637,0.00540364639161632,
0.00540659419243178,0.00630457583191594,0.00630769322450373,0.00675524744892423,
0.00675824274053971,0.00698081395851806,0.0069835174985577,0.00709382875298428,
0.00709615487756669,0.00715056271684698,0.00715247356707119,0.00717033207045985,
0.00717923745439373,0.00718063291182344,0.00719131802773085,0.00720628339444832,
0.00720879225482352),.UNSPECIFIED.);
#988=B_SPLINE_CURVE_WITH_KNOTS('',3,(#31442,#31443,#31444,#31445,#31446,
#31447,#31448,#31449,#31450,#31451,#31452,#31453,#31454,#31455,#31456,#31457,
#31458,#31459,#31460,#31461,#31462,#31463,#31464,#31465,#31466,#31467,#31468,
#31469,#31470,#31471,#31472,#31473,#31474,#31475,#31476,#31477,#31478,#31479,
#31480,#31481,#31482,#31483,#31484,#31485,#31486,#31487,#31488,#31489,#31490,
#31491,#31492,#31493,#31494,#31495,#31496,#31497,#31498,#31499,#31500,#31501,
#31502,#31503,#31504,#31505,#31506,#31507,#31508,#31509,#31510,#31511,#31512,
#31513,#31514,#31515,#31516,#31517),.UNSPECIFIED.,.F.,.F.,(4,3,3,3,3,3,
3,3,3,3,3,3,3,3,3,3,3,3,3,3,3,3,3,3,3,4),(1.92266797596103E-13,0.000100765253400692,
0.000203257746196736,0.000307659288333143,0.000415034136597425,0.000522822845455063,
0.000628818251273869,0.000674714477361159,0.000796110490146888,0.000926752228731723,
0.00108084544056301,0.00125483099502789,0.00134942895472221,0.00150980300002335,
0.0016863707781532,0.00182669577876767,0.00195048914404132,0.00202414343208326,
0.00212087565257403,0.00221840926324827,0.00231581884120266,0.00236150067076378,
0.00246857997997598,0.00257529118717096,0.00268062322103986,0.00269885790944431),
 .UNSPECIFIED.);
#989=B_SPLINE_CURVE_WITH_KNOTS('',3,(#31746,#31747,#31748,#31749,#31750,
#31751,#31752,#31753,#31754,#31755,#31756,#31757,#31758,#31759,#31760,#31761,
#31762,#31763,#31764,#31765,#31766,#31767,#31768,#31769,#31770,#31771,#31772,
#31773,#31774,#31775,#31776,#31777,#31778,#31779,#31780,#31781,#31782,#31783,
#31784,#31785,#31786,#31787,#31788,#31789,#31790,#31791,#31792,#31793,#31794,
#31795,#31796,#31797,#31798,#31799,#31800,#31801,#31802,#31803,#31804,#31805,
#31806,#31807,#31808,#31809,#31810,#31811,#31812,#31813,#31814,#31815,#31816,
#31817,#31818,#31819,#31820,#31821),.UNSPECIFIED.,.F.,.F.,(4,3,3,3,3,3,
3,3,3,3,3,3,3,3,3,3,3,3,3,3,3,3,3,3,3,4),(6.6900740202938E-10,0.000100568281496774,
0.000202839043311474,0.000306975484988691,0.000413993960739299,0.000521383938195942,
0.000626986625570161,0.000674714477360893,0.000795619140822781,0.000925351564806097,
0.00108316358964099,0.00125449955005232,0.0013494289547216,0.00150400641422797,
0.00167742957890143,0.0018187480346269,0.00194314871130111,0.00202414343208231,
0.00212118997393239,0.002219037980227,0.00231672327406803,0.00236150067076266,
0.00246941783078403,0.00257682685345429,0.00268261453841891,0.00269885790944302),
 .UNSPECIFIED.);
#1025=CONICAL_SURFACE('',#18059,7.85653654166145,0.904103500540624);
#1026=CONICAL_SURFACE('',#18079,12.25,0.118705337143177);
#1119=SHAPE_REPRESENTATION_RELATIONSHIP('SRR','None',#38692,#1133);
#1133=ADVANCED_BREP_SHAPE_REPRESENTATION('',(#1179),#38628);
#1153=STYLED_ITEM('',(#38767),#1179);
#1179=MANIFOLD_SOLID_BREP('Body1',#17619);
#1255=PLANE('',#18088);
#1256=PLANE('',#18089);
#1257=PLANE('',#18091);
#1258=PLANE('',#18100);
#1259=PLANE('',#18102);
#1808=FACE_OUTER_BOUND('',#2827,.T.);
#1809=FACE_OUTER_BOUND('',#2828,.T.);
#1810=FACE_OUTER_BOUND('',#2829,.T.);
#1811=FACE_OUTER_BOUND('',#2830,.T.);
#1812=FACE_OUTER_BOUND('',#2831,.T.);
#1813=FACE_OUTER_BOUND('',#2832,.T.);
#1814=FACE_OUTER_BOUND('',#2833,.T.);
#1815=FACE_OUTER_BOUND('',#2834,.T.);
#1816=FACE_OUTER_BOUND('',#2835,.T.);
#1817=FACE_OUTER_BOUND('',#2836,.T.);
#1818=FACE_OUTER_BOUND('',#2838,.T.);
#1819=FACE_OUTER_BOUND('',#2839,.T.);
#1820=FACE_OUTER_BOUND('',#2840,.T.);
#1821=FACE_OUTER_BOUND('',#2841,.T.);
#1822=FACE_OUTER_BOUND('',#2842,.T.);
#1823=FACE_OUTER_BOUND('',#2843,.T.);
#1824=FACE_OUTER_BOUND('',#2844,.T.);
#1825=FACE_OUTER_BOUND('',#2845,.T.);
#1826=FACE_OUTER_BOUND('',#2846,.T.);
#1827=FACE_OUTER_BOUND('',#2847,.T.);
#1828=FACE_OUTER_BOUND('',#2848,.T.);
#1829=FACE_OUTER_BOUND('',#2849,.T.);
#1830=FACE_OUTER_BOUND('',#2850,.T.);
#1831=FACE_OUTER_BOUND('',#2851,.T.);
#1832=FACE_OUTER_BOUND('',#2852,.T.);
#1833=FACE_OUTER_BOUND('',#2853,.T.);
#1834=FACE_OUTER_BOUND('',#2854,.T.);
#1835=FACE_OUTER_BOUND('',#2855,.T.);
#1836=FACE_OUTER_BOUND('',#2856,.T.);
#1837=FACE_OUTER_BOUND('',#2857,.T.);
#1838=FACE_OUTER_BOUND('',#2858,.T.);
#1839=FACE_OUTER_BOUND('',#2859,.T.);
#1840=FACE_OUTER_BOUND('',#2860,.T.);
#1841=FACE_OUTER_BOUND('',#2861,.T.);
#1842=FACE_OUTER_BOUND('',#2862,.T.);
#2827=EDGE_LOOP('',(#11701,#11702,#11703,#11704));
#2828=EDGE_LOOP('',(#11705,#11706,#11707));
#2829=EDGE_LOOP('',(#11708,#11709,#11710,#11711));
#2830=EDGE_LOOP('',(#11712,#11713,#11714,#11715,#11716,#11717));
#2831=EDGE_LOOP('',(#11718,#11719,#11720,#11721));
#2832=EDGE_LOOP('',(#11722,#11723,#11724,#11725,#11726,#11727,#11728,#11729,
#11730));
#2833=EDGE_LOOP('',(#11731,#11732,#11733,#11734,#11735,#11736,#11737,#11738,
#11739));
#2834=EDGE_LOOP('',(#11740,#11741,#11742,#11743,#11744,#11745,#11746));
#2835=EDGE_LOOP('',(#11747,#11748,#11749,#11750,#11751,#11752,#11753,#11754));
#2836=EDGE_LOOP('',(#11755));
#2837=EDGE_LOOP('',(#11756));
#2838=EDGE_LOOP('',(#11757,#11758,#11759));
#2839=EDGE_LOOP('',(#11760,#11761,#11762));
#2840=EDGE_LOOP('',(#11763,#11764,#11765,#11766,#11767,#11768,#11769,#11770,
#11771,#11772,#11773,#11774,#11775,#11776,#11777));
#2841=EDGE_LOOP('',(#11778,#11779,#11780,#11781));
#2842=EDGE_LOOP('',(#11782,#11783,#11784,#11785));
#2843=EDGE_LOOP('',(#11786,#11787,#11788));
#2844=EDGE_LOOP('',(#11789,#11790,#11791));
#2845=EDGE_LOOP('',(#11792,#11793,#11794));
#2846=EDGE_LOOP('',(#11795,#11796,#11797,#11798));
#2847=EDGE_LOOP('',(#11799,#11800,#11801,#11802));
#2848=EDGE_LOOP('',(#11803,#11804,#11805));
#2849=EDGE_LOOP('',(#11806,#11807,#11808,#11809));
#2850=EDGE_LOOP('',(#11810,#11811,#11812));
#2851=EDGE_LOOP('',(#11813,#11814,#11815,#11816));
#2852=EDGE_LOOP('',(#11817,#11818,#11819));
#2853=EDGE_LOOP('',(#11820,#11821,#11822,#11823,#11824));
#2854=EDGE_LOOP('',(#11825,#11826,#11827,#11828,#11829));
#2855=EDGE_LOOP('',(#11830,#11831,#11832,#11833,#11834));
#2856=EDGE_LOOP('',(#11835,#11836,#11837));
#2857=EDGE_LOOP('',(#11838,#11839,#11840,#11841));
#2858=EDGE_LOOP('',(#11842,#11843,#11844,#11845));
#2859=EDGE_LOOP('',(#11846,#11847,#11848));
#2860=EDGE_LOOP('',(#11849,#11850,#11851,#11852));
#2861=EDGE_LOOP('',(#11853,#11854,#11855,#11856));
#2862=EDGE_LOOP('',(#11857,#11858,#11859,#11860));
#3884=LINE('',#29983,#4828);
#3885=LINE('',#30000,#4829);
#3886=LINE('',#30025,#4830);
#3887=LINE('',#30446,#4831);
#3888=LINE('',#30628,#4832);
#3889=LINE('',#30641,#4833);
#3890=LINE('',#30654,#4834);
#3891=LINE('',#30767,#4835);
#3892=LINE('',#31044,#4836);
#3893=LINE('',#31240,#4837);
#3894=LINE('',#31246,#4838);
#3895=LINE('',#31251,#4839);
#3896=LINE('',#31253,#4840);
#4828=VECTOR('',#20477,7.85653654166145);
#4829=VECTOR('',#20498,1000.);
#4830=VECTOR('',#20501,1000.);
#4831=VECTOR('',#20520,12.25);
#4832=VECTOR('',#20533,1000.);
#4833=VECTOR('',#20534,6.);
#4834=VECTOR('',#20537,1000.);
#4835=VECTOR('',#20550,1000.);
#4836=VECTOR('',#20551,1000.);
#4837=VECTOR('',#20556,1000.);
#4838=VECTOR('',#20563,1000.);
#4839=VECTOR('',#20570,1000.);
#4840=VECTOR('',#20573,1000.);
#5686=CIRCLE('',#18060,9.11842675485531);
#5687=CIRCLE('',#18061,7.85653654166145);
#5688=CIRCLE('',#18063,1.);
#5689=CIRCLE('',#18064,1.);
#5690=CIRCLE('',#18065,0.999999999999999);
#5691=CIRCLE('',#18067,6.);
#5692=CIRCLE('',#18068,0.999999999999998);
#5693=CIRCLE('',#18069,7.62222222222222);
#5694=CIRCLE('',#18071,6.);
#5695=CIRCLE('',#18073,6.57777777777778);
#5696=CIRCLE('',#18075,9.25);
#5697=CIRCLE('',#18076,9.25);
#5698=CIRCLE('',#18077,6.);
#5699=CIRCLE('',#18078,9.25);
#5700=CIRCLE('',#18080,12.25);
#5701=CIRCLE('',#18081,12.25);
#5702=CIRCLE('',#18084,10.3623383247004);
#5703=CIRCLE('',#18085,10.3623383247004);
#5704=CIRCLE('',#18087,6.);
#5705=CIRCLE('',#18090,9.25);
#5706=CIRCLE('',#18092,9.25);
#5707=CIRCLE('',#18095,1.);
#5708=CIRCLE('',#18096,1.);
#5709=CIRCLE('',#18098,1.);
#5710=CIRCLE('',#18099,1.);
#5711=CIRCLE('',#18101,9.51643315533714);
#5712=CIRCLE('',#18103,9.51643315533713);
#5713=CIRCLE('',#18104,1.);
#5714=CIRCLE('',#18105,1.);
#5715=CIRCLE('',#18106,1.);
#5716=CIRCLE('',#18108,1.);
#5717=CIRCLE('',#18110,1.);
#5718=CIRCLE('',#18112,1.);
#5719=CIRCLE('',#18114,1.);
#5720=CIRCLE('',#18116,1.);
#5721=CIRCLE('',#18117,1.);
#5722=CIRCLE('',#18119,1.);
#5723=CIRCLE('',#18122,1.);
#5724=CIRCLE('',#18124,1.);
#5725=CIRCLE('',#18125,1.);
#5726=CIRCLE('',#18126,1.);
#6774=VERTEX_POINT('',#29980);
#6775=VERTEX_POINT('',#29982);
#6776=VERTEX_POINT('',#29986);
#6777=VERTEX_POINT('',#29987);
#6778=VERTEX_POINT('',#29989);
#6779=VERTEX_POINT('',#29993);
#6780=VERTEX_POINT('',#29995);
#6781=VERTEX_POINT('',#29999);
#6782=VERTEX_POINT('',#30001);
#6783=VERTEX_POINT('',#30012);
#6784=VERTEX_POINT('',#30014);
#6785=VERTEX_POINT('',#30027);
#6786=VERTEX_POINT('',#30028);
#6787=VERTEX_POINT('',#30159);
#6788=VERTEX_POINT('',#30227);
#6789=VERTEX_POINT('',#30295);
#6790=VERTEX_POINT('',#30297);
#6791=VERTEX_POINT('',#30302);
#6792=VERTEX_POINT('',#30304);
#6793=VERTEX_POINT('',#30308);
#6794=VERTEX_POINT('',#30309);
#6795=VERTEX_POINT('',#30437);
#6796=VERTEX_POINT('',#30444);
#6797=VERTEX_POINT('',#30447);
#6798=VERTEX_POINT('',#30449);
#6799=VERTEX_POINT('',#30594);
#6800=VERTEX_POINT('',#30610);
#6801=VERTEX_POINT('',#30627);
#6802=VERTEX_POINT('',#30629);
#6803=VERTEX_POINT('',#30640);
#6804=VERTEX_POINT('',#30643);
#6805=VERTEX_POINT('',#30661);
#6806=VERTEX_POINT('',#30741);
#6807=VERTEX_POINT('',#30758);
#6808=VERTEX_POINT('',#30766);
#6809=VERTEX_POINT('',#30768);
#6810=VERTEX_POINT('',#30783);
#6811=VERTEX_POINT('',#31028);
#6812=VERTEX_POINT('',#31043);
#6813=VERTEX_POINT('',#31045);
#6814=VERTEX_POINT('',#31053);
#6815=VERTEX_POINT('',#31237);
#6816=VERTEX_POINT('',#31239);
#6817=VERTEX_POINT('',#31243);
#6818=VERTEX_POINT('',#31245);
#6819=VERTEX_POINT('',#31249);
#8637=EDGE_CURVE('',#6774,#6774,#5686,.T.);
#8638=EDGE_CURVE('',#6774,#6775,#3884,.T.);
#8639=EDGE_CURVE('',#6775,#6775,#5687,.T.);
#8640=EDGE_CURVE('',#6776,#6777,#5688,.T.);
#8641=EDGE_CURVE('',#6778,#6777,#5689,.T.);
#8642=EDGE_CURVE('',#6776,#6778,#5690,.T.);
#8643=EDGE_CURVE('',#6778,#6779,#5691,.T.);
#8644=EDGE_CURVE('',#6779,#6780,#5692,.T.);
#8645=EDGE_CURVE('',#6776,#6780,#5693,.T.);
#8646=EDGE_CURVE('',#6778,#6781,#3885,.T.);
#8647=EDGE_CURVE('',#6781,#6782,#965,.T.);
#8648=EDGE_CURVE('',#6782,#6783,#5694,.T.);
#8649=EDGE_CURVE('',#6783,#6784,#966,.T.);
#8650=EDGE_CURVE('',#6784,#6779,#3886,.T.);
#8651=EDGE_CURVE('',#6785,#6786,#5695,.T.);
#8652=EDGE_CURVE('',#6786,#6783,#967,.T.);
#8653=EDGE_CURVE('',#6782,#6785,#968,.T.);
#8654=EDGE_CURVE('',#6787,#6786,#969,.T.);
#8655=EDGE_CURVE('',#6785,#6788,#970,.T.);
#8656=EDGE_CURVE('',#6789,#6788,#5696,.T.);
#8657=EDGE_CURVE('',#6788,#6790,#971,.T.);
#8658=EDGE_CURVE('',#6791,#6790,#5697,.T.);
#8659=EDGE_CURVE('',#6791,#6792,#5698,.T.);
#8660=EDGE_CURVE('',#6787,#6792,#5699,.T.);
#8661=EDGE_CURVE('',#6793,#6794,#972,.T.);
#8662=EDGE_CURVE('',#6794,#6795,#973,.T.);
#8663=EDGE_CURVE('',#6795,#6796,#5700,.T.);
#8664=EDGE_CURVE('',#6796,#6774,#3887,.T.);
#8665=EDGE_CURVE('',#6796,#6797,#5701,.T.);
#8666=EDGE_CURVE('',#6797,#6798,#67,.T.);
#8667=EDGE_CURVE('',#6798,#6793,#974,.T.);
#8668=EDGE_CURVE('',#6780,#6799,#5702,.T.);
#8669=EDGE_CURVE('',#6799,#6797,#975,.T.);
#8670=EDGE_CURVE('',#6795,#6800,#976,.T.);
#8671=EDGE_CURVE('',#6800,#6776,#5703,.T.);
#8672=EDGE_CURVE('',#6801,#6791,#3888,.T.);
#8673=EDGE_CURVE('',#6801,#6802,#977,.T.);
#8674=EDGE_CURVE('',#6802,#6803,#3889,.T.);
#8675=EDGE_CURVE('',#6803,#6803,#5704,.T.);
#8676=EDGE_CURVE('',#6802,#6804,#978,.T.);
#8677=EDGE_CURVE('',#6792,#6804,#3890,.T.);
#8678=EDGE_CURVE('',#6801,#6790,#5705,.T.);
#8679=EDGE_CURVE('',#6787,#6804,#5706,.T.);
#8680=EDGE_CURVE('',#6790,#6805,#979,.T.);
#8681=EDGE_CURVE('',#6805,#6806,#980,.T.);
#8682=EDGE_CURVE('',#6806,#6807,#981,.T.);
#8683=EDGE_CURVE('',#6808,#6807,#3891,.T.);
#8684=EDGE_CURVE('',#6808,#6809,#982,.T.);
#8685=EDGE_CURVE('',#6809,#6810,#983,.T.);
#8686=EDGE_CURVE('',#6810,#6811,#984,.T.);
#8687=EDGE_CURVE('',#6811,#6812,#3892,.T.);
#8688=EDGE_CURVE('',#6812,#6813,#985,.T.);
#8689=EDGE_CURVE('',#6813,#6814,#986,.T.);
#8690=EDGE_CURVE('',#6814,#6787,#987,.T.);
#8691=EDGE_CURVE('',#6807,#6815,#5707,.T.);
#8692=EDGE_CURVE('',#6816,#6815,#3893,.T.);
#8693=EDGE_CURVE('',#6816,#6808,#5708,.T.);
#8694=EDGE_CURVE('',#6811,#6817,#5709,.T.);
#8695=EDGE_CURVE('',#6817,#6818,#3894,.T.);
#8696=EDGE_CURVE('',#6818,#6812,#5710,.T.);
#8697=EDGE_CURVE('',#6817,#6819,#5711,.T.);
#8698=EDGE_CURVE('',#6819,#6818,#3895,.T.);
#8699=EDGE_CURVE('',#6815,#6777,#3896,.T.);
#8700=EDGE_CURVE('',#6777,#6816,#5712,.T.);
#8701=EDGE_CURVE('',#6786,#6814,#5713,.T.);
#8702=EDGE_CURVE('',#6783,#6813,#5714,.T.);
#8703=EDGE_CURVE('',#6784,#6812,#5715,.T.);
#8704=EDGE_CURVE('',#6784,#6818,#5716,.T.);
#8705=EDGE_CURVE('',#6779,#6819,#5717,.T.);
#8706=EDGE_CURVE('',#6780,#6819,#5718,.T.);
#8707=EDGE_CURVE('',#6799,#6817,#5719,.T.);
#8708=EDGE_CURVE('',#6799,#6811,#5720,.T.);
#8709=EDGE_CURVE('',#6798,#6810,#988,.T.);
#8710=EDGE_CURVE('',#6794,#6809,#989,.T.);
#8711=EDGE_CURVE('',#6800,#6808,#5721,.T.);
#8712=EDGE_CURVE('',#6800,#6816,#5722,.T.);
#8713=EDGE_CURVE('',#6781,#6815,#5723,.T.);
#8714=EDGE_CURVE('',#6781,#6807,#5724,.T.);
#8715=EDGE_CURVE('',#6782,#6806,#5725,.T.);
#8716=EDGE_CURVE('',#6785,#6805,#5726,.T.);
#11701=ORIENTED_EDGE('',*,*,#8637,.F.);
#11702=ORIENTED_EDGE('',*,*,#8638,.T.);
#11703=ORIENTED_EDGE('',*,*,#8639,.F.);
#11704=ORIENTED_EDGE('',*,*,#8638,.F.);
#11705=ORIENTED_EDGE('',*,*,#8640,.T.);
#11706=ORIENTED_EDGE('',*,*,#8641,.F.);
#11707=ORIENTED_EDGE('',*,*,#8642,.F.);
#11708=ORIENTED_EDGE('',*,*,#8643,.T.);
#11709=ORIENTED_EDGE('',*,*,#8644,.T.);
#11710=ORIENTED_EDGE('',*,*,#8645,.F.);
#11711=ORIENTED_EDGE('',*,*,#8642,.T.);
#11712=ORIENTED_EDGE('',*,*,#8643,.F.);
#11713=ORIENTED_EDGE('',*,*,#8646,.T.);
#11714=ORIENTED_EDGE('',*,*,#8647,.T.);
#11715=ORIENTED_EDGE('',*,*,#8648,.T.);
#11716=ORIENTED_EDGE('',*,*,#8649,.T.);
#11717=ORIENTED_EDGE('',*,*,#8650,.T.);
#11718=ORIENTED_EDGE('',*,*,#8651,.T.);
#11719=ORIENTED_EDGE('',*,*,#8652,.T.);
#11720=ORIENTED_EDGE('',*,*,#8648,.F.);
#11721=ORIENTED_EDGE('',*,*,#8653,.T.);
#11722=ORIENTED_EDGE('',*,*,#8654,.T.);
#11723=ORIENTED_EDGE('',*,*,#8651,.F.);
#11724=ORIENTED_EDGE('',*,*,#8655,.T.);
#11725=ORIENTED_EDGE('',*,*,#8656,.F.);
#11726=ORIENTED_EDGE('',*,*,#8656,.T.);
#11727=ORIENTED_EDGE('',*,*,#8657,.T.);
#11728=ORIENTED_EDGE('',*,*,#8658,.F.);
#11729=ORIENTED_EDGE('',*,*,#8659,.T.);
#11730=ORIENTED_EDGE('',*,*,#8660,.F.);
#11731=ORIENTED_EDGE('',*,*,#8661,.T.);
#11732=ORIENTED_EDGE('',*,*,#8662,.T.);
#11733=ORIENTED_EDGE('',*,*,#8663,.T.);
#11734=ORIENTED_EDGE('',*,*,#8664,.T.);
#11735=ORIENTED_EDGE('',*,*,#8637,.T.);
#11736=ORIENTED_EDGE('',*,*,#8664,.F.);
#11737=ORIENTED_EDGE('',*,*,#8665,.T.);
#11738=ORIENTED_EDGE('',*,*,#8666,.T.);
#11739=ORIENTED_EDGE('',*,*,#8667,.T.);
#11740=ORIENTED_EDGE('',*,*,#8645,.T.);
#11741=ORIENTED_EDGE('',*,*,#8668,.T.);
#11742=ORIENTED_EDGE('',*,*,#8669,.T.);
#11743=ORIENTED_EDGE('',*,*,#8665,.F.);
#11744=ORIENTED_EDGE('',*,*,#8663,.F.);
#11745=ORIENTED_EDGE('',*,*,#8670,.T.);
#11746=ORIENTED_EDGE('',*,*,#8671,.T.);
#11747=ORIENTED_EDGE('',*,*,#8659,.F.);
#11748=ORIENTED_EDGE('',*,*,#8672,.F.);
#11749=ORIENTED_EDGE('',*,*,#8673,.T.);
#11750=ORIENTED_EDGE('',*,*,#8674,.T.);
#11751=ORIENTED_EDGE('',*,*,#8675,.T.);
#11752=ORIENTED_EDGE('',*,*,#8674,.F.);
#11753=ORIENTED_EDGE('',*,*,#8676,.T.);
#11754=ORIENTED_EDGE('',*,*,#8677,.F.);
#11755=ORIENTED_EDGE('',*,*,#8639,.T.);
#11756=ORIENTED_EDGE('',*,*,#8675,.F.);
#11757=ORIENTED_EDGE('',*,*,#8672,.T.);
#11758=ORIENTED_EDGE('',*,*,#8658,.T.);
#11759=ORIENTED_EDGE('',*,*,#8678,.F.);
#11760=ORIENTED_EDGE('',*,*,#8677,.T.);
#11761=ORIENTED_EDGE('',*,*,#8679,.F.);
#11762=ORIENTED_EDGE('',*,*,#8660,.T.);
#11763=ORIENTED_EDGE('',*,*,#8678,.T.);
#11764=ORIENTED_EDGE('',*,*,#8680,.T.);
#11765=ORIENTED_EDGE('',*,*,#8681,.T.);
#11766=ORIENTED_EDGE('',*,*,#8682,.T.);
#11767=ORIENTED_EDGE('',*,*,#8683,.F.);
#11768=ORIENTED_EDGE('',*,*,#8684,.T.);
#11769=ORIENTED_EDGE('',*,*,#8685,.T.);
#11770=ORIENTED_EDGE('',*,*,#8686,.T.);
#11771=ORIENTED_EDGE('',*,*,#8687,.T.);
#11772=ORIENTED_EDGE('',*,*,#8688,.T.);
#11773=ORIENTED_EDGE('',*,*,#8689,.T.);
#11774=ORIENTED_EDGE('',*,*,#8690,.T.);
#11775=ORIENTED_EDGE('',*,*,#8679,.T.);
#11776=ORIENTED_EDGE('',*,*,#8676,.F.);
#11777=ORIENTED_EDGE('',*,*,#8673,.F.);
#11778=ORIENTED_EDGE('',*,*,#8683,.T.);
#11779=ORIENTED_EDGE('',*,*,#8691,.T.);
#11780=ORIENTED_EDGE('',*,*,#8692,.F.);
#11781=ORIENTED_EDGE('',*,*,#8693,.T.);
#11782=ORIENTED_EDGE('',*,*,#8687,.F.);
#11783=ORIENTED_EDGE('',*,*,#8694,.T.);
#11784=ORIENTED_EDGE('',*,*,#8695,.T.);
#11785=ORIENTED_EDGE('',*,*,#8696,.T.);
#11786=ORIENTED_EDGE('',*,*,#8695,.F.);
#11787=ORIENTED_EDGE('',*,*,#8697,.T.);
#11788=ORIENTED_EDGE('',*,*,#8698,.T.);
#11789=ORIENTED_EDGE('',*,*,#8692,.T.);
#11790=ORIENTED_EDGE('',*,*,#8699,.T.);
#11791=ORIENTED_EDGE('',*,*,#8700,.T.);
#11792=ORIENTED_EDGE('',*,*,#8690,.F.);
#11793=ORIENTED_EDGE('',*,*,#8701,.F.);
#11794=ORIENTED_EDGE('',*,*,#8654,.F.);
#11795=ORIENTED_EDGE('',*,*,#8701,.T.);
#11796=ORIENTED_EDGE('',*,*,#8689,.F.);
#11797=ORIENTED_EDGE('',*,*,#8702,.F.);
#11798=ORIENTED_EDGE('',*,*,#8652,.F.);
#11799=ORIENTED_EDGE('',*,*,#8702,.T.);
#11800=ORIENTED_EDGE('',*,*,#8688,.F.);
#11801=ORIENTED_EDGE('',*,*,#8703,.F.);
#11802=ORIENTED_EDGE('',*,*,#8649,.F.);
#11803=ORIENTED_EDGE('',*,*,#8703,.T.);
#11804=ORIENTED_EDGE('',*,*,#8696,.F.);
#11805=ORIENTED_EDGE('',*,*,#8704,.F.);
#11806=ORIENTED_EDGE('',*,*,#8705,.F.);
#11807=ORIENTED_EDGE('',*,*,#8650,.F.);
#11808=ORIENTED_EDGE('',*,*,#8704,.T.);
#11809=ORIENTED_EDGE('',*,*,#8698,.F.);
#11810=ORIENTED_EDGE('',*,*,#8644,.F.);
#11811=ORIENTED_EDGE('',*,*,#8705,.T.);
#11812=ORIENTED_EDGE('',*,*,#8706,.F.);
#11813=ORIENTED_EDGE('',*,*,#8706,.T.);
#11814=ORIENTED_EDGE('',*,*,#8697,.F.);
#11815=ORIENTED_EDGE('',*,*,#8707,.F.);
#11816=ORIENTED_EDGE('',*,*,#8668,.F.);
#11817=ORIENTED_EDGE('',*,*,#8707,.T.);
#11818=ORIENTED_EDGE('',*,*,#8694,.F.);
#11819=ORIENTED_EDGE('',*,*,#8708,.F.);
#11820=ORIENTED_EDGE('',*,*,#8708,.T.);
#11821=ORIENTED_EDGE('',*,*,#8686,.F.);
#11822=ORIENTED_EDGE('',*,*,#8709,.F.);
#11823=ORIENTED_EDGE('',*,*,#8666,.F.);
#11824=ORIENTED_EDGE('',*,*,#8669,.F.);
#11825=ORIENTED_EDGE('',*,*,#8709,.T.);
#11826=ORIENTED_EDGE('',*,*,#8685,.F.);
#11827=ORIENTED_EDGE('',*,*,#8710,.F.);
#11828=ORIENTED_EDGE('',*,*,#8661,.F.);
#11829=ORIENTED_EDGE('',*,*,#8667,.F.);
#11830=ORIENTED_EDGE('',*,*,#8710,.T.);
#11831=ORIENTED_EDGE('',*,*,#8684,.F.);
#11832=ORIENTED_EDGE('',*,*,#8711,.F.);
#11833=ORIENTED_EDGE('',*,*,#8670,.F.);
#11834=ORIENTED_EDGE('',*,*,#8662,.F.);
#11835=ORIENTED_EDGE('',*,*,#8711,.T.);
#11836=ORIENTED_EDGE('',*,*,#8693,.F.);
#11837=ORIENTED_EDGE('',*,*,#8712,.F.);
#11838=ORIENTED_EDGE('',*,*,#8640,.F.);
#11839=ORIENTED_EDGE('',*,*,#8671,.F.);
#11840=ORIENTED_EDGE('',*,*,#8712,.T.);
#11841=ORIENTED_EDGE('',*,*,#8700,.F.);
#11842=ORIENTED_EDGE('',*,*,#8641,.T.);
#11843=ORIENTED_EDGE('',*,*,#8699,.F.);
#11844=ORIENTED_EDGE('',*,*,#8713,.F.);
#11845=ORIENTED_EDGE('',*,*,#8646,.F.);
#11846=ORIENTED_EDGE('',*,*,#8713,.T.);
#11847=ORIENTED_EDGE('',*,*,#8691,.F.);
#11848=ORIENTED_EDGE('',*,*,#8714,.F.);
#11849=ORIENTED_EDGE('',*,*,#8714,.T.);
#11850=ORIENTED_EDGE('',*,*,#8682,.F.);
#11851=ORIENTED_EDGE('',*,*,#8715,.F.);
#11852=ORIENTED_EDGE('',*,*,#8647,.F.);
#11853=ORIENTED_EDGE('',*,*,#8715,.T.);
#11854=ORIENTED_EDGE('',*,*,#8681,.F.);
#11855=ORIENTED_EDGE('',*,*,#8716,.F.);
#11856=ORIENTED_EDGE('',*,*,#8653,.F.);
#11857=ORIENTED_EDGE('',*,*,#8655,.F.);
#11858=ORIENTED_EDGE('',*,*,#8716,.T.);
#11859=ORIENTED_EDGE('',*,*,#8680,.F.);
#11860=ORIENTED_EDGE('',*,*,#8657,.F.);
#16332=CYLINDRICAL_SURFACE('',#18070,6.);
#16333=CYLINDRICAL_SURFACE('',#18086,6.);
#16334=CYLINDRICAL_SURFACE('',#18093,9.25);
#16335=CYLINDRICAL_SURFACE('',#18094,1.);
#16336=CYLINDRICAL_SURFACE('',#18097,1.);
#16337=CYLINDRICAL_SURFACE('',#18109,1.);
#16338=CYLINDRICAL_SURFACE('',#18121,1.);
#16767=ADVANCED_FACE('',(#1808),#1025,.T.);
#16768=ADVANCED_FACE('',(#1809),#79,.T.);
#16769=ADVANCED_FACE('',(#1810),#145,.T.);
#16770=ADVANCED_FACE('',(#1811),#16332,.F.);
#16771=ADVANCED_FACE('',(#1812),#146,.T.);
#16772=ADVANCED_FACE('',(#1813),#80,.F.);
#16773=ADVANCED_FACE('',(#1814),#1026,.T.);
#16774=ADVANCED_FACE('',(#1815),#81,.T.);
#16775=ADVANCED_FACE('',(#1816),#16333,.F.);
#16776=ADVANCED_FACE('',(#1817,#875),#1255,.F.);
#16777=ADVANCED_FACE('',(#1818),#1256,.T.);
#16778=ADVANCED_FACE('',(#1819),#1257,.T.);
#16779=ADVANCED_FACE('',(#1820),#16334,.F.);
#16780=ADVANCED_FACE('',(#1821),#16335,.T.);
#16781=ADVANCED_FACE('',(#1822),#16336,.T.);
#16782=ADVANCED_FACE('',(#1823),#1258,.F.);
#16783=ADVANCED_FACE('',(#1824),#1259,.F.);
#16784=ADVANCED_FACE('',(#1825),#126,.T.);
#16785=ADVANCED_FACE('',(#1826),#127,.T.);
#16786=ADVANCED_FACE('',(#1827),#128,.T.);
#16787=ADVANCED_FACE('',(#1828),#82,.T.);
#16788=ADVANCED_FACE('',(#1829),#16337,.T.);
#16789=ADVANCED_FACE('',(#1830),#83,.T.);
#16790=ADVANCED_FACE('',(#1831),#147,.T.);
#16791=ADVANCED_FACE('',(#1832),#84,.T.);
#16792=ADVANCED_FACE('',(#1833),#129,.T.);
#16793=ADVANCED_FACE('',(#1834),#130,.T.);
#16794=ADVANCED_FACE('',(#1835),#131,.T.);
#16795=ADVANCED_FACE('',(#1836),#85,.T.);
#16796=ADVANCED_FACE('',(#1837),#148,.T.);
#16797=ADVANCED_FACE('',(#1838),#16338,.T.);
#16798=ADVANCED_FACE('',(#1839),#86,.T.);
#16799=ADVANCED_FACE('',(#1840),#132,.T.);
#16800=ADVANCED_FACE('',(#1841),#133,.T.);
#16801=ADVANCED_FACE('',(#1842),#134,.T.);
#17619=CLOSED_SHELL('',(#16767,#16768,#16769,#16770,#16771,#16772,#16773,
#16774,#16775,#16776,#16777,#16778,#16779,#16780,#16781,#16782,#16783,#16784,
#16785,#16786,#16787,#16788,#16789,#16790,#16791,#16792,#16793,#16794,#16795,
#16796,#16797,#16798,#16799,#16800,#16801));
#18058=AXIS2_PLACEMENT_3D('',#29978,#20471,#20472);
#18059=AXIS2_PLACEMENT_3D('',#29979,#20473,#20474);
#18060=AXIS2_PLACEMENT_3D('',#29981,#20475,#20476);
#18061=AXIS2_PLACEMENT_3D('',#29984,#20478,#20479);
#18062=AXIS2_PLACEMENT_3D('',#29985,#20480,#20481);
#18063=AXIS2_PLACEMENT_3D('',#29988,#20482,#20483);
#18064=AXIS2_PLACEMENT_3D('',#29990,#20484,#20485);
#18065=AXIS2_PLACEMENT_3D('',#29991,#20486,#20487);
#18066=AXIS2_PLACEMENT_3D('',#29992,#20488,#20489);
#18067=AXIS2_PLACEMENT_3D('',#29994,#20490,#20491);
#18068=AXIS2_PLACEMENT_3D('',#29996,#20492,#20493);
#18069=AXIS2_PLACEMENT_3D('',#29997,#20494,#20495);
#18070=AXIS2_PLACEMENT_3D('',#29998,#20496,#20497);
#18071=AXIS2_PLACEMENT_3D('',#30013,#20499,#20500);
#18072=AXIS2_PLACEMENT_3D('',#30026,#20502,#20503);
#18073=AXIS2_PLACEMENT_3D('',#30029,#20504,#20505);
#18074=AXIS2_PLACEMENT_3D('',#30158,#20506,#20507);
#18075=AXIS2_PLACEMENT_3D('',#30296,#20508,#20509);
#18076=AXIS2_PLACEMENT_3D('',#30303,#20510,#20511);
#18077=AXIS2_PLACEMENT_3D('',#30305,#20512,#20513);
#18078=AXIS2_PLACEMENT_3D('',#30306,#20514,#20515);
#18079=AXIS2_PLACEMENT_3D('',#30307,#20516,#20517);
#18080=AXIS2_PLACEMENT_3D('',#30445,#20518,#20519);
#18081=AXIS2_PLACEMENT_3D('',#30448,#20521,#20522);
#18082=AXIS2_PLACEMENT_3D('',#30450,#20523,#20524);
#18083=AXIS2_PLACEMENT_3D('',#30593,#20525,#20526);
#18084=AXIS2_PLACEMENT_3D('',#30595,#20527,#20528);
#18085=AXIS2_PLACEMENT_3D('',#30625,#20529,#20530);
#18086=AXIS2_PLACEMENT_3D('',#30626,#20531,#20532);
#18087=AXIS2_PLACEMENT_3D('',#30642,#20535,#20536);
#18088=AXIS2_PLACEMENT_3D('',#30655,#20538,#20539);
#18089=AXIS2_PLACEMENT_3D('',#30656,#20540,#20541);
#18090=AXIS2_PLACEMENT_3D('',#30657,#20542,#20543);
#18091=AXIS2_PLACEMENT_3D('',#30658,#20544,#20545);
#18092=AXIS2_PLACEMENT_3D('',#30659,#20546,#20547);
#18093=AXIS2_PLACEMENT_3D('',#30660,#20548,#20549);
#18094=AXIS2_PLACEMENT_3D('',#31236,#20552,#20553);
#18095=AXIS2_PLACEMENT_3D('',#31238,#20554,#20555);
#18096=AXIS2_PLACEMENT_3D('',#31241,#20557,#20558);
#18097=AXIS2_PLACEMENT_3D('',#31242,#20559,#20560);
#18098=AXIS2_PLACEMENT_3D('',#31244,#20561,#20562);
#18099=AXIS2_PLACEMENT_3D('',#31247,#20564,#20565);
#18100=AXIS2_PLACEMENT_3D('',#31248,#20566,#20567);
#18101=AXIS2_PLACEMENT_3D('',#31250,#20568,#20569);
#18102=AXIS2_PLACEMENT_3D('',#31252,#20571,#20572);
#18103=AXIS2_PLACEMENT_3D('',#31254,#20574,#20575);
#18104=AXIS2_PLACEMENT_3D('',#31327,#20576,#20577);
#18105=AXIS2_PLACEMENT_3D('',#31376,#20578,#20579);
#18106=AXIS2_PLACEMENT_3D('',#31389,#20580,#20581);
#18107=AXIS2_PLACEMENT_3D('',#31390,#20582,#20583);
#18108=AXIS2_PLACEMENT_3D('',#31391,#20584,#20585);
#18109=AXIS2_PLACEMENT_3D('',#31392,#20586,#20587);
#18110=AXIS2_PLACEMENT_3D('',#31393,#20588,#20589);
#18111=AXIS2_PLACEMENT_3D('',#31394,#20590,#20591);
#18112=AXIS2_PLACEMENT_3D('',#31395,#20592,#20593);
#18113=AXIS2_PLACEMENT_3D('',#31396,#20594,#20595);
#18114=AXIS2_PLACEMENT_3D('',#31397,#20596,#20597);
#18115=AXIS2_PLACEMENT_3D('',#31398,#20598,#20599);
#18116=AXIS2_PLACEMENT_3D('',#31399,#20600,#20601);
#18117=AXIS2_PLACEMENT_3D('',#31864,#20602,#20603);
#18118=AXIS2_PLACEMENT_3D('',#31865,#20604,#20605);
#18119=AXIS2_PLACEMENT_3D('',#31866,#20606,#20607);
#18120=AXIS2_PLACEMENT_3D('',#31867,#20608,#20609);
#18121=AXIS2_PLACEMENT_3D('',#31868,#20610,#20611);
#18122=AXIS2_PLACEMENT_3D('',#31869,#20612,#20613);
#18123=AXIS2_PLACEMENT_3D('',#31870,#20614,#20615);
#18124=AXIS2_PLACEMENT_3D('',#31871,#20616,#20617);
#18125=AXIS2_PLACEMENT_3D('',#31884,#20618,#20619);
#18126=AXIS2_PLACEMENT_3D('',#31927,#20620,#20621);
#20471=DIRECTION('axis',(0.,0.,1.));
#20472=DIRECTION('refdir',(1.,0.,0.));
#20473=DIRECTION('center_axis',(1.,0.,0.));
#20474=DIRECTION('ref_axis',(0.,0.,-1.));
#20475=DIRECTION('center_axis',(1.,0.,0.));
#20476=DIRECTION('ref_axis',(0.,0.,1.));
#20477=DIRECTION('',(-0.618390361344798,9.62414507819028E-17,-0.785871084209013));
#20478=DIRECTION('center_axis',(-1.,0.,0.));
#20479=DIRECTION('ref_axis',(0.,0.,-1.));
#20480=DIRECTION('center_axis',(0.,0.,1.));
#20481=DIRECTION('ref_axis',(1.,8.88178419700125E-16,0.));
#20482=DIRECTION('center_axis',(0.378876330722911,-1.20404638253675E-15,
0.925447311313801));
#20483=DIRECTION('ref_axis',(0.925447311313801,1.02297272535146E-30,-0.378876330722911));
#20484=DIRECTION('center_axis',(-1.,1.16846812913649E-29,-1.34715203352919E-14));
#20485=DIRECTION('ref_axis',(-1.34715203352919E-14,-4.74710593547472E-45,
1.));
#20486=DIRECTION('center_axis',(0.,-0.515078753637713,0.857142857142857));
#20487=DIRECTION('ref_axis',(0.,-0.857142857142857,-0.515078753637713));
#20488=DIRECTION('center_axis',(-1.,0.,0.));
#20489=DIRECTION('ref_axis',(0.,0.,1.));
#20490=DIRECTION('center_axis',(-1.,0.,0.));
#20491=DIRECTION('ref_axis',(0.,0.,1.));
#20492=DIRECTION('center_axis',(0.,0.515078753637713,0.857142857142857));
#20493=DIRECTION('ref_axis',(0.,0.857142857142857,-0.515078753637713));
#20494=DIRECTION('center_axis',(-1.,0.,0.));
#20495=DIRECTION('ref_axis',(0.,0.,1.));
#20496=DIRECTION('center_axis',(-1.,0.,0.));
#20497=DIRECTION('ref_axis',(0.,0.,1.));
#20498=DIRECTION('',(-1.,0.,0.));
#20499=DIRECTION('center_axis',(-1.,0.,0.));
#20500=DIRECTION('ref_axis',(0.,0.,1.));
#20501=DIRECTION('',(1.,0.,0.));
#20502=DIRECTION('center_axis',(-1.,0.,0.));
#20503=DIRECTION('ref_axis',(0.,0.,1.));
#20504=DIRECTION('center_axis',(-1.,0.,0.));
#20505=DIRECTION('ref_axis',(0.,0.,1.));
#20506=DIRECTION('center_axis',(0.,6.12323399573677E-17,-1.));
#20507=DIRECTION('ref_axis',(0.,1.,0.));
#20508=DIRECTION('center_axis',(1.,0.,0.));
#20509=DIRECTION('ref_axis',(0.,-1.,0.));
#20510=DIRECTION('center_axis',(0.,0.,1.));
#20511=DIRECTION('ref_axis',(-1.,0.,0.));
#20512=DIRECTION('center_axis',(-1.,0.,0.));
#20513=DIRECTION('ref_axis',(0.,0.,1.));
#20514=DIRECTION('center_axis',(0.,0.,1.));
#20515=DIRECTION('ref_axis',(-1.,-1.77635683940025E-15,0.));
#20516=DIRECTION('center_axis',(1.,0.,0.));
#20517=DIRECTION('ref_axis',(0.,0.,-1.));
#20518=DIRECTION('center_axis',(-1.,0.,0.));
#20519=DIRECTION('ref_axis',(0.,0.,1.));
#20520=DIRECTION('',(-0.992962790709924,1.45030946266966E-17,-0.118426754855312));
#20521=DIRECTION('center_axis',(-1.,0.,0.));
#20522=DIRECTION('ref_axis',(0.,0.,1.));
#20523=DIRECTION('center_axis',(-0.129239030503541,0.903475790448336,-0.408691532905026));
#20524=DIRECTION('ref_axis',(0.134650954949434,0.42432007345752,0.895444914884333));
#20525=DIRECTION('center_axis',(1.,-3.74939945665464E-33,6.12323399573677E-17));
#20526=DIRECTION('ref_axis',(0.,-6.12323399573677E-17,1.));
#20527=DIRECTION('center_axis',(0.,1.,0.));
#20528=DIRECTION('ref_axis',(1.87495354061429E-14,0.,-1.));
#20529=DIRECTION('center_axis',(7.01804016390762E-16,-1.,0.));
#20530=DIRECTION('ref_axis',(-1.,-7.01804016390762E-16,1.06581410364015E-14));
#20531=DIRECTION('center_axis',(-1.,0.,0.));
#20532=DIRECTION('ref_axis',(0.,0.,1.));
#20533=DIRECTION('',(1.,0.,0.));
#20534=DIRECTION('',(-1.,0.,0.));
#20535=DIRECTION('center_axis',(-1.,0.,0.));
#20536=DIRECTION('ref_axis',(0.,0.,1.));
#20537=DIRECTION('',(-1.,0.,0.));
#20538=DIRECTION('center_axis',(1.,0.,0.));
#20539=DIRECTION('ref_axis',(0.,0.,-1.));
#20540=DIRECTION('center_axis',(0.,0.,-1.));
#20541=DIRECTION('ref_axis',(-1.,0.,0.));
#20542=DIRECTION('center_axis',(0.,0.,1.));
#20543=DIRECTION('ref_axis',(1.,0.,0.));
#20544=DIRECTION('center_axis',(0.,0.,-1.));
#20545=DIRECTION('ref_axis',(-1.,0.,0.));
#20546=DIRECTION('center_axis',(0.,0.,1.));
#20547=DIRECTION('ref_axis',(1.,0.,0.));
#20548=DIRECTION('center_axis',(0.,0.,1.));
#20549=DIRECTION('ref_axis',(-1.,7.6571373978539E-16,0.));
#20550=DIRECTION('',(0.,0.,1.));
#20551=DIRECTION('',(0.,0.,1.));
#20552=DIRECTION('center_axis',(0.,0.,1.));
#20553=DIRECTION('ref_axis',(1.,0.,0.));
#20554=DIRECTION('center_axis',(0.,0.,-1.));
#20555=DIRECTION('ref_axis',(1.,4.33680868994201E-15,0.));
#20556=DIRECTION('',(0.,0.,1.));
#20557=DIRECTION('center_axis',(0.,0.,1.));
#20558=DIRECTION('ref_axis',(1.,0.,0.));
#20559=DIRECTION('center_axis',(0.,0.,1.));
#20560=DIRECTION('ref_axis',(1.,0.,0.));
#20561=DIRECTION('center_axis',(0.,0.,1.));
#20562=DIRECTION('ref_axis',(1.,0.,0.));
#20563=DIRECTION('',(0.,0.,1.));
#20564=DIRECTION('center_axis',(0.,0.,-1.));
#20565=DIRECTION('ref_axis',(1.,-2.60208521396521E-15,0.));
#20566=DIRECTION('center_axis',(0.,1.,0.));
#20567=DIRECTION('ref_axis',(0.,0.,1.));
#20568=DIRECTION('center_axis',(0.,-1.,0.));
#20569=DIRECTION('ref_axis',(-6.9269116917139E-15,0.,1.));
#20570=DIRECTION('',(-1.,0.,0.));
#20571=DIRECTION('center_axis',(7.01804016390762E-16,-1.,0.));
#20572=DIRECTION('ref_axis',(1.,7.01804016390762E-16,0.));
#20573=DIRECTION('',(1.,7.01804016390762E-16,0.));
#20574=DIRECTION('center_axis',(-7.01804016390762E-16,1.,0.));
#20575=DIRECTION('ref_axis',(1.,7.01804016390762E-16,0.));
#20576=DIRECTION('center_axis',(0.709785481558855,-0.704116397237294,-0.020607506152819));
#20577=DIRECTION('ref_axis',(0.704265953185076,0.709936241633231,4.28924729850355E-17));
#20578=DIRECTION('center_axis',(0.29037131728916,-0.353646401377125,-0.889167431302321));
#20579=DIRECTION('ref_axis',(-7.39118707684208E-18,0.929203026942477,-0.369569661526671));
#20580=DIRECTION('center_axis',(0.348558970379625,-0.482776543868745,-0.803388730850791));
#20581=DIRECTION('ref_axis',(-1.8398092574652E-17,0.857142857142857,-0.515078753637713));
#20582=DIRECTION('center_axis',(1.,0.,0.));
#20583=DIRECTION('ref_axis',(0.,0.515078753637713,0.857142857142857));
#20584=DIRECTION('center_axis',(1.,0.,0.));
#20585=DIRECTION('ref_axis',(0.,0.,-1.));
#20586=DIRECTION('center_axis',(-1.,0.,0.));
#20587=DIRECTION('ref_axis',(0.,0.,1.));
#20588=DIRECTION('center_axis',(1.,6.93889390390723E-15,1.15470174302502E-14));
#20589=DIRECTION('ref_axis',(1.15470174302502E-14,-1.61729683642884E-29,
-1.));
#20590=DIRECTION('center_axis',(0.,0.,1.));
#20591=DIRECTION('ref_axis',(1.,0.,0.));
#20592=DIRECTION('center_axis',(-0.378876330722912,4.01348794178917E-16,
-0.925447311313801));
#20593=DIRECTION('ref_axis',(-0.925447311313801,1.31246556823689E-31,0.378876330722912));
#20594=DIRECTION('center_axis',(0.,1.,0.));
#20595=DIRECTION('ref_axis',(0.,0.,1.));
#20596=DIRECTION('center_axis',(-0.489525396383285,0.,-0.871989040238343));
#20597=DIRECTION('ref_axis',(-0.871989040238343,0.,0.489525396383285));
#20598=DIRECTION('center_axis',(1.,0.,0.));
#20599=DIRECTION('ref_axis',(0.,-1.,0.));
#20600=DIRECTION('center_axis',(-0.585365170384224,0.810768328674619,0.00152791335295939));
#20601=DIRECTION('ref_axis',(-0.810769275053396,-0.585365853658539,-3.50084822314998E-20));
#20602=DIRECTION('center_axis',(0.58536517038422,0.810768328674621,-0.00152791335296999));
#20603=DIRECTION('ref_axis',(-0.810769275053399,0.585365853658535,-2.27653634851535E-20));
#20604=DIRECTION('center_axis',(1.,0.,0.));
#20605=DIRECTION('ref_axis',(0.,-1.,0.));
#20606=DIRECTION('center_axis',(0.489525396383287,0.,0.871989040238343));
#20607=DIRECTION('ref_axis',(0.871989040238342,0.,-0.489525396383287));
#20608=DIRECTION('center_axis',(7.01804016390762E-16,-1.,0.));
#20609=DIRECTION('ref_axis',(1.,7.60106174710418E-16,0.));
#20610=DIRECTION('center_axis',(-1.,0.,0.));
#20611=DIRECTION('ref_axis',(0.,0.,1.));
#20612=DIRECTION('center_axis',(-1.,0.,0.));
#20613=DIRECTION('ref_axis',(0.,0.,1.));
#20614=DIRECTION('center_axis',(1.,0.,0.));
#20615=DIRECTION('ref_axis',(0.,0.515078753637712,-0.857142857142858));
#20616=DIRECTION('center_axis',(-0.348558970379622,-0.482776543868745,0.803388730850793));
#20617=DIRECTION('ref_axis',(2.32069397924157E-17,-0.857142857142857,-0.515078753637712));
#20618=DIRECTION('center_axis',(-0.29037131728916,-0.353646401377124,0.889167431302321));
#20619=DIRECTION('ref_axis',(-4.59831187317044E-17,-0.929203026942477,-0.369569661526671));
#20620=DIRECTION('center_axis',(-0.709785481558847,-0.7041163972373,0.0206075061528517));
#20621=DIRECTION('ref_axis',(0.704265953185083,-0.709936241633223,2.61261679533882E-17));
#29978=CARTESIAN_POINT('',(0.,0.,0.));
#29979=CARTESIAN_POINT('Origin',(-3.88784034431744,0.,0.));
#29980=CARTESIAN_POINT('',(-2.89487755360751,-1.11668521385931E-15,9.11842675485531));
#29981=CARTESIAN_POINT('Origin',(-2.89487755360751,0.,0.));
#29982=CARTESIAN_POINT('',(-3.88784034431744,-9.62148232812991E-16,7.85653654166145));
#29983=CARTESIAN_POINT('',(-3.88784034431744,-9.62148232812991E-16,7.85653654166145));
#29984=CARTESIAN_POINT('Origin',(-3.88784034431744,0.,0.));
#29985=CARTESIAN_POINT('Origin',(32.1691171325868,-6.,-3.60555127546399));
#29986=CARTESIAN_POINT('',(32.9519577972005,-6.53333333333333,-3.9260447221719));
#29987=CARTESIAN_POINT('',(32.1691171325868,-5.,-3.60555127546399));
#29988=CARTESIAN_POINT('Origin',(32.1691171325868,-6.,-3.60555127546399));
#29989=CARTESIAN_POINT('',(32.1691171325868,-5.14285714285715,-3.09047252182628));
#29990=CARTESIAN_POINT('Origin',(32.1691171325868,-6.,-3.60555127546399));
#29991=CARTESIAN_POINT('Origin',(32.1691171325868,-6.,-3.60555127546399));
#29992=CARTESIAN_POINT('Origin',(32.1691171325868,0.,0.));
#29993=CARTESIAN_POINT('',(32.1691171325868,5.14285714285714,-3.09047252182628));
#29994=CARTESIAN_POINT('Origin',(32.1691171325868,0.,0.));
#29995=CARTESIAN_POINT('',(32.9519577972005,6.53333333333333,-3.9260447221719));
#29996=CARTESIAN_POINT('Origin',(32.1691171325868,6.,-3.60555127546399));
#29997=CARTESIAN_POINT('Origin',(32.9519577972005,0.,0.));
#29998=CARTESIAN_POINT('Origin',(-60.4312629272455,0.,0.));
#29999=CARTESIAN_POINT('',(31.6603850692973,-5.1428571428572,-3.09047252182618));
#30000=CARTESIAN_POINT('',(-60.4312629272455,-5.1428571428572,-3.09047252182618));
#30001=CARTESIAN_POINT('',(31.2718056654608,-5.57521816165486,-2.21741796916002));
#30002=CARTESIAN_POINT('Ctrl Pts',(31.6603850692973,-5.1428571428572,-3.09047252182618));
#30003=CARTESIAN_POINT('Ctrl Pts',(31.6130789304298,-5.19901889001868,-2.99701372531371));
#30004=CARTESIAN_POINT('Ctrl Pts',(31.566662826541,-5.25269307059619,-2.90193250281435));
#30005=CARTESIAN_POINT('Ctrl Pts',(31.5214090737152,-5.30390019323349,-2.80511011195956));
#30006=CARTESIAN_POINT('Ctrl Pts',(31.4766400999664,-5.35455876154984,-2.70932492722243));
#30007=CARTESIAN_POINT('Ctrl Pts',(31.4330087073867,-5.40280302228635,-2.61183520986889));
#30008=CARTESIAN_POINT('Ctrl Pts',(31.3907785539495,-5.4486054329858,-2.51250847473946));
#30009=CARTESIAN_POINT('Ctrl Pts',(31.3497152496182,-5.49314229057631,-2.41592620778376));
#30010=CARTESIAN_POINT('Ctrl Pts',(31.3099768197504,-5.53537039074759,-2.3176065755272));
#30011=CARTESIAN_POINT('Ctrl Pts',(31.2718056654607,-5.57521816165486,-2.21741796916003));
#30012=CARTESIAN_POINT('',(31.2718056654608,5.57521816165486,-2.21741796916003));
#30013=CARTESIAN_POINT('Origin',(31.2718056654608,0.,0.));
#30014=CARTESIAN_POINT('',(31.6603850692973,5.14285714285714,-3.09047252182628));
#30015=CARTESIAN_POINT('Ctrl Pts',(31.2718056654607,5.57521816165486,-2.21741796916003));
#30016=CARTESIAN_POINT('Ctrl Pts',(31.3109482377269,5.53435630454291,-2.32015627608185));
#30017=CARTESIAN_POINT('Ctrl Pts',(31.3517388718349,5.49099163463111,-2.42092930418135));
#30018=CARTESIAN_POINT('Ctrl Pts',(31.3939161850971,5.44520068393954,-2.51987886844277));
#30019=CARTESIAN_POINT('Ctrl Pts',(31.436608060703,5.39885108460289,-2.62003561532806));
#30020=CARTESIAN_POINT('Ctrl Pts',(31.4807206567692,5.35001548035485,-2.71832462698763));
#30021=CARTESIAN_POINT('Ctrl Pts',(31.5259829068312,5.29872070791517,-2.81488167771062));
#30022=CARTESIAN_POINT('Ctrl Pts',(31.5697886823089,5.24907652801694,-2.90833166039983));
#30023=CARTESIAN_POINT('Ctrl Pts',(31.6146713137554,5.197128415931,-3.00015966435589));
#30024=CARTESIAN_POINT('Ctrl Pts',(31.6603850692973,5.14285714285714,-3.09047252182628));
#30025=CARTESIAN_POINT('',(-60.4312629272455,5.14285714285714,-3.09047252182628));
#30026=CARTESIAN_POINT('Origin',(31.2718056654608,0.,0.));
#30027=CARTESIAN_POINT('',(29.8656463748335,-6.5669102351073,-0.377955629499295));
#30028=CARTESIAN_POINT('',(29.8656463748335,6.5669102351073,-0.377955629499269));
#30029=CARTESIAN_POINT('Origin',(29.8656463748335,0.,0.));
#30030=CARTESIAN_POINT('Ctrl Pts',(29.8656463748335,6.56691023510728,-0.377955629499269));
#30031=CARTESIAN_POINT('Ctrl Pts',(29.8725075439928,6.5601223945667,-0.377832908785134));
#30032=CARTESIAN_POINT('Ctrl Pts',(29.8790313233221,6.55371594181744,-0.378533417250872));
#30033=CARTESIAN_POINT('Ctrl Pts',(29.8852810759567,6.54761680930762,-0.379843594119964));
#30034=CARTESIAN_POINT('Ctrl Pts',(29.8918523561381,6.54120389812085,-0.381221174929515));
#30035=CARTESIAN_POINT('Ctrl Pts',(29.8981209111568,6.53513071591201,-0.3832764131639));
#30036=CARTESIAN_POINT('Ctrl Pts',(29.9041291486039,6.52934354017054,-0.385782549958447));
#30037=CARTESIAN_POINT('Ctrl Pts',(29.9075083267445,6.52608869248297,-0.387192061940608));
#30038=CARTESIAN_POINT('Ctrl Pts',(29.9108045893958,6.52292489077237,-0.388744297301114));
#30039=CARTESIAN_POINT('Ctrl Pts',(29.9140210253342,6.51984677993087,-0.39039428080563));
#30040=CARTESIAN_POINT('Ctrl Pts',(29.9204153242607,6.51372747234116,-0.393674460468415));
#30041=CARTESIAN_POINT('Ctrl Pts',(29.9265008152716,6.50793946229219,-0.397332941703034));
#30042=CARTESIAN_POINT('Ctrl Pts',(29.9324249507833,6.50233824792647,-0.401361685578881));
#30043=CARTESIAN_POINT('Ctrl Pts',(29.9373301272236,6.49770044977186,-0.404697480228541));
#30044=CARTESIAN_POINT('Ctrl Pts',(29.9421235535095,6.49319187366407,-0.40828778998665));
#30045=CARTESIAN_POINT('Ctrl Pts',(29.9469087678782,6.48871046304552,-0.41211279361687));
#30046=CARTESIAN_POINT('Ctrl Pts',(29.9479028070629,6.48777953343309,-0.412907366899729));
#30047=CARTESIAN_POINT('Ctrl Pts',(29.9488966014781,6.48684966489765,-0.413711988676514));
#30048=CARTESIAN_POINT('Ctrl Pts',(29.9498912775077,6.48591974131433,-0.414526339789525));
#30049=CARTESIAN_POINT('Ctrl Pts',(29.9576241534814,6.47869026807829,-0.42085732190663));
#30050=CARTESIAN_POINT('Ctrl Pts',(29.9654019249319,6.47146767959501,-0.427811739749593));
#30051=CARTESIAN_POINT('Ctrl Pts',(29.9733209196286,6.46417108245538,-0.435510985707953));
#30052=CARTESIAN_POINT('Ctrl Pts',(29.9829182505443,6.45532805881548,-0.44484199476825));
#30053=CARTESIAN_POINT('Ctrl Pts',(29.9919885021345,6.44705359857573,-0.454544762727445));
#30054=CARTESIAN_POINT('Ctrl Pts',(30.0008134547635,6.43906208798889,-0.464442747702182));
#30055=CARTESIAN_POINT('Ctrl Pts',(30.0025614062969,6.43747921567539,-0.466403233921351));
#30056=CARTESIAN_POINT('Ctrl Pts',(30.0042998323013,6.43590734417065,-0.468371296570632));
#30057=CARTESIAN_POINT('Ctrl Pts',(30.0060310804752,6.4343440929234,-0.470345432705976));
#30058=CARTESIAN_POINT('Ctrl Pts',(30.0191369783573,6.42250996566295,-0.485290041447687));
#30059=CARTESIAN_POINT('Ctrl Pts',(30.031839751297,6.41116861900765,-0.500703061129736));
#30060=CARTESIAN_POINT('Ctrl Pts',(30.0443550852513,6.40011900637697,-0.516607199583796));
#30061=CARTESIAN_POINT('Ctrl Pts',(30.0506060384155,6.39460012759283,-0.52455073708397));
#30062=CARTESIAN_POINT('Ctrl Pts',(30.0568106516791,6.38915364007045,-0.532616634573869));
#30063=CARTESIAN_POINT('Ctrl Pts',(30.0629994771853,6.38375101060815,-0.540806413681568));
#30064=CARTESIAN_POINT('Ctrl Pts',(30.0748370591151,6.37341721321275,-0.556471289202405));
#30065=CARTESIAN_POINT('Ctrl Pts',(30.0864049630046,6.36342886769562,-0.572310950518507));
#30066=CARTESIAN_POINT('Ctrl Pts',(30.0979191698185,6.35357062888264,-0.588245141470827));
#30067=CARTESIAN_POINT('Ctrl Pts',(30.1211338537217,6.3336946702878,-0.620371297635091));
#30068=CARTESIAN_POINT('Ctrl Pts',(30.1439826702986,6.31449626551089,-0.652929314975647));
#30069=CARTESIAN_POINT('Ctrl Pts',(30.166659015077,6.29578657510829,-0.685777462655701));
#30070=CARTESIAN_POINT('Ctrl Pts',(30.1868553837943,6.27912305152682,-0.715033205091633));
#30071=CARTESIAN_POINT('Ctrl Pts',(30.2069158355587,6.26284623933258,-0.744518847551107));
#30072=CARTESIAN_POINT('Ctrl Pts',(30.2269993156952,6.24679677088334,-0.774128879324885));
#30073=CARTESIAN_POINT('Ctrl Pts',(30.2389447497761,6.23725072278359,-0.791740602008511));
#30074=CARTESIAN_POINT('Ctrl Pts',(30.2508989662365,6.22778417331905,-0.809398803531555));
#30075=CARTESIAN_POINT('Ctrl Pts',(30.2629011553761,6.21835795433208,-0.827084782242122));
#30076=CARTESIAN_POINT('Ctrl Pts',(30.302268731467,6.18743964527177,-0.885095375520649));
#30077=CARTESIAN_POINT('Ctrl Pts',(30.3420024626169,6.15710898525446,-0.943463646964114));
#30078=CARTESIAN_POINT('Ctrl Pts',(30.3821258030208,6.12732774116849,-1.00198727566907));
#30079=CARTESIAN_POINT('Ctrl Pts',(30.4277433739611,6.09346844627666,-1.06852475129435));
#30080=CARTESIAN_POINT('Ctrl Pts',(30.4738648259364,6.06031882234849,-1.1352629705455));
#30081=CARTESIAN_POINT('Ctrl Pts',(30.5205608459579,6.02776378653948,-1.20191078358617));
#30082=CARTESIAN_POINT('Ctrl Pts',(30.5330992620028,6.01902238666983,-1.21980648450457));
#30083=CARTESIAN_POINT('Ctrl Pts',(30.5456792644843,6.01032359736377,-1.23769570207054));
#30084=CARTESIAN_POINT('Ctrl Pts',(30.5583025227219,6.00166470917368,-1.25557287713379));
#30085=CARTESIAN_POINT('Ctrl Pts',(30.5681724071966,5.99489448990794,-1.26955069880942));
#30086=CARTESIAN_POINT('Ctrl Pts',(30.5780684551723,5.98814840962004,-1.28352288344113));
#30087=CARTESIAN_POINT('Ctrl Pts',(30.5879926334101,5.98142414590736,-1.29748907624301));
#30088=CARTESIAN_POINT('Ctrl Pts',(30.6669544011375,5.92792251215015,-1.40861115059904));
#30089=CARTESIAN_POINT('Ctrl Pts',(30.7475298903906,5.87599870594709,-1.51939708458653));
#30090=CARTESIAN_POINT('Ctrl Pts',(30.8293107323995,5.82574321254352,-1.63008315076544));
#30091=CARTESIAN_POINT('Ctrl Pts',(30.9214154700563,5.76914353807153,-1.75474206643868));
#30092=CARTESIAN_POINT('Ctrl Pts',(31.0150485279702,5.71466041937621,-1.87927598022933));
#30093=CARTESIAN_POINT('Ctrl Pts',(31.1095944938123,5.66237027343985,-2.0040523816082));
#30094=CARTESIAN_POINT('Ctrl Pts',(31.1634082906049,5.63260769962077,-2.07507277733319));
#30095=CARTESIAN_POINT('Ctrl Pts',(31.2175173246529,5.60355460236516,-2.14617211425946));
#30096=CARTESIAN_POINT('Ctrl Pts',(31.2718056654608,5.57521816165486,-2.21741796916003));
#30097=CARTESIAN_POINT('Ctrl Pts',(31.2718056654608,-5.57521816165487,-2.21741796916002));
#30098=CARTESIAN_POINT('Ctrl Pts',(31.1819875314053,-5.62209979760386,-2.09954422960071));
#30099=CARTESIAN_POINT('Ctrl Pts',(31.0927465664112,-5.67089537566277,-1.98218339393731));
#30100=CARTESIAN_POINT('Ctrl Pts',(31.0046065204154,-5.72156004652258,-1.86503220805667));
#30101=CARTESIAN_POINT('Ctrl Pts',(30.9255422977669,-5.76700775161531,-1.75994413668838));
#30102=CARTESIAN_POINT('Ctrl Pts',(30.8473642922524,-5.81395915530375,-1.65502294282812));
#30103=CARTESIAN_POINT('Ctrl Pts',(30.7704327542947,-5.86234777851516,-1.55005512612116));
#30104=CARTESIAN_POINT('Ctrl Pts',(30.7086828848192,-5.90118739158838,-1.46580165670074));
#30105=CARTESIAN_POINT('Ctrl Pts',(30.6477358551072,-5.94095238471506,-1.38151794451207));
#30106=CARTESIAN_POINT('Ctrl Pts',(30.5877661622583,-5.98159134441235,-1.29710698186777));
#30107=CARTESIAN_POINT('Ctrl Pts',(30.5783243505759,-5.98798966640143,-1.28381706198719));
#30108=CARTESIAN_POINT('Ctrl Pts',(30.5689093564766,-5.99440681250476,-1.27052356904323));
#30109=CARTESIAN_POINT('Ctrl Pts',(30.5595195554009,-6.00084470060566,-1.25722696506484));
#30110=CARTESIAN_POINT('Ctrl Pts',(30.5031524419472,-6.03949143721509,-1.17740725653641));
#30111=CARTESIAN_POINT('Ctrl Pts',(30.4476477085009,-6.0789178589505,-1.09741768380242));
#30112=CARTESIAN_POINT('Ctrl Pts',(30.3926547385931,-6.1195304846082,-1.01734187625657));
#30113=CARTESIAN_POINT('Ctrl Pts',(30.3490261759155,-6.15175042993903,-0.953813894510328));
#30114=CARTESIAN_POINT('Ctrl Pts',(30.3057199242426,-6.18471646153748,-0.890231728104117));
#30115=CARTESIAN_POINT('Ctrl Pts',(30.2625722572727,-6.21861100640185,-0.826639841079345));
#30116=CARTESIAN_POINT('Ctrl Pts',(30.2509982419382,-6.22770294600282,-0.809581827813351));
#30117=CARTESIAN_POINT('Ctrl Pts',(30.2394493761657,-6.23684780069786,-0.792518945606304));
#30118=CARTESIAN_POINT('Ctrl Pts',(30.227886703887,-6.24608463641092,-0.77546319513685));
#30119=CARTESIAN_POINT('Ctrl Pts',(30.2052208675914,-6.26419122986221,-0.742029501028785));
#30120=CARTESIAN_POINT('Ctrl Pts',(30.182685244376,-6.28250490217154,-0.708903832679339));
#30121=CARTESIAN_POINT('Ctrl Pts',(30.1600108241324,-6.30128103849979,-0.676163278587289));
#30122=CARTESIAN_POINT('Ctrl Pts',(30.1393594431902,-6.31838194515021,-0.646343876479036));
#30123=CARTESIAN_POINT('Ctrl Pts',(30.1185934610269,-6.3358659017507,-0.616843789210932));
#30124=CARTESIAN_POINT('Ctrl Pts',(30.097535297881,-6.35389930559972,-0.587714258355697));
#30125=CARTESIAN_POINT('Ctrl Pts',(30.086119151503,-6.36367565582589,-0.571922425712827));
#30126=CARTESIAN_POINT('Ctrl Pts',(30.0746477525123,-6.37358221414102,-0.556221757231938));
#30127=CARTESIAN_POINT('Ctrl Pts',(30.0629107652948,-6.38382864590174,-0.54069175867353));
#30128=CARTESIAN_POINT('Ctrl Pts',(30.0534369671071,-6.39209930555624,-0.528156338001143));
#30129=CARTESIAN_POINT('Ctrl Pts',(30.043919380635,-6.40047911568583,-0.51590652917707));
#30130=CARTESIAN_POINT('Ctrl Pts',(30.0343494281368,-6.4089793588288,-0.504052250919162));
#30131=CARTESIAN_POINT('Ctrl Pts',(30.0254564440403,-6.4168783036879,-0.493036531871049));
#30132=CARTESIAN_POINT('Ctrl Pts',(30.0165182973371,-6.4248811549012,-0.482362363619343));
#30133=CARTESIAN_POINT('Ctrl Pts',(30.007561954601,-6.43296147857311,-0.472106200546239));
#30134=CARTESIAN_POINT('Ctrl Pts',(30.0068801630943,-6.43357658411489,-0.471325461679847));
#30135=CARTESIAN_POINT('Ctrl Pts',(30.0061982830898,-6.43419212095116,-0.470547139131873));
#30136=CARTESIAN_POINT('Ctrl Pts',(30.0055163349455,-6.4348080686191,-0.469771263647443));
#30137=CARTESIAN_POINT('Ctrl Pts',(29.999426485346,-6.4403085288674,-0.462842635645629));
#30138=CARTESIAN_POINT('Ctrl Pts',(29.9933391033403,-6.44583328872601,-0.456096771562847));
#30139=CARTESIAN_POINT('Ctrl Pts',(29.987190434343,-6.45144755712158,-0.449605478393239));
#30140=CARTESIAN_POINT('Ctrl Pts',(29.9834438098157,-6.45486855045898,-0.44565007955589));
#30141=CARTESIAN_POINT('Ctrl Pts',(29.9796750763159,-6.45832211622899,-0.441788848226876));
#30142=CARTESIAN_POINT('Ctrl Pts',(29.9758760317652,-6.46181664631018,-0.438034612133003));
#30143=CARTESIAN_POINT('Ctrl Pts',(29.9672827168783,-6.46972115939749,-0.42954265251402));
#30144=CARTESIAN_POINT('Ctrl Pts',(29.9585336198971,-6.47783579642184,-0.421599175152793));
#30145=CARTESIAN_POINT('Ctrl Pts',(29.9494315602762,-6.48634799335753,-0.414175830172066));
#30146=CARTESIAN_POINT('Ctrl Pts',(29.9443612126388,-6.49108975504875,-0.410040618884511));
#30147=CARTESIAN_POINT('Ctrl Pts',(29.9391527039694,-6.49597193326323,-0.405860302400109));
#30148=CARTESIAN_POINT('Ctrl Pts',(29.9337071438672,-6.50110604110052,-0.401902571557844));
#30149=CARTESIAN_POINT('Ctrl Pts',(29.927097252935,-6.50733788726545,-0.397098626928533));
#30150=CARTESIAN_POINT('Ctrl Pts',(29.9201388905088,-6.51394006959045,-0.392621605951022));
#30151=CARTESIAN_POINT('Ctrl Pts',(29.9126651940782,-6.5210985400584,-0.38887619517018));
#30152=CARTESIAN_POINT('Ctrl Pts',(29.9048166960573,-6.52861600371532,-0.384942954186471));
#30153=CARTESIAN_POINT('Ctrl Pts',(29.8964014607698,-6.53674516224513,-0.381812401352293));
#30154=CARTESIAN_POINT('Ctrl Pts',(29.8872163718764,-6.54571003340667,-0.379924022087368));
#30155=CARTESIAN_POINT('Ctrl Pts',(29.8804719643197,-6.55229273995512,-0.378537426973039));
#30156=CARTESIAN_POINT('Ctrl Pts',(29.8733123700361,-6.55932610303385,-0.377819678470141));
#30157=CARTESIAN_POINT('Ctrl Pts',(29.8656463748432,-6.56691023509677,-0.377955629499085));
#30158=CARTESIAN_POINT('Origin',(23.3621596556826,0.,0.));
#30159=CARTESIAN_POINT('',(23.3560798022767,9.24999809463599,-6.60452283141046E-10));
#30160=CARTESIAN_POINT('Ctrl Pts',(23.3560798282383,9.24999837277875,-6.67384040739516E-9));
#30161=CARTESIAN_POINT('Ctrl Pts',(23.3566780177678,9.24999837572821,-0.0102225537292777));
#30162=CARTESIAN_POINT('Ctrl Pts',(23.3670051565122,9.24999029805898,-0.0157301067324773));
#30163=CARTESIAN_POINT('Ctrl Pts',(23.375414584291,9.24996826963113,-0.0202809688865867));
#30164=CARTESIAN_POINT('Ctrl Pts',(23.3754183438715,9.24996825978294,-0.0202830034284274));
#30165=CARTESIAN_POINT('Ctrl Pts',(23.3754221035694,9.24996824993205,-0.0202850377621649));
#30166=CARTESIAN_POINT('Ctrl Pts',(23.3754258633847,9.24996824007846,-0.0202870718878598));
#30167=CARTESIAN_POINT('Ctrl Pts',(23.3838350809832,9.24994620151217,-0.0248366054593298));
#30168=CARTESIAN_POINT('Ctrl Pts',(23.3928310844359,9.24991067376018,-0.0283456960327398));
#30169=CARTESIAN_POINT('Ctrl Pts',(23.4018732133928,9.2498611248735,-0.0314960934238296));
#30170=CARTESIAN_POINT('Ctrl Pts',(23.401878048676,9.24986109837721,-0.0314977781005028));
#30171=CARTESIAN_POINT('Ctrl Pts',(23.401882883983,9.24986107187696,-0.0314994626675972));
#30172=CARTESIAN_POINT('Ctrl Pts',(23.4018877193138,9.24986104537276,-0.0315011471251339));
#30173=CARTESIAN_POINT('Ctrl Pts',(23.4199770283062,9.24976189130746,-0.0378028200424206));
#30174=CARTESIAN_POINT('Ctrl Pts',(23.4383987060992,9.24960739037706,-0.0425720268385514));
#30175=CARTESIAN_POINT('Ctrl Pts',(23.4569145494441,9.24939573886127,-0.0469039022173839));
#30176=CARTESIAN_POINT('Ctrl Pts',(23.4569194598224,9.24939568273156,-0.0469050510252594));
#30177=CARTESIAN_POINT('Ctrl Pts',(23.4569243702082,9.24939562659782,-0.0469061997977794));
#30178=CARTESIAN_POINT('Ctrl Pts',(23.4569292806017,9.24939557046007,-0.0469073485349474));
#30179=CARTESIAN_POINT('Ctrl Pts',(23.4939660705805,9.24897214978062,-0.0555717330220713));
#30180=CARTESIAN_POINT('Ctrl Pts',(23.5314364698805,9.2483200844845,-0.0622254714305722));
#30181=CARTESIAN_POINT('Ctrl Pts',(23.569035993724,9.24743432044532,-0.0682690984893951));
#30182=CARTESIAN_POINT('Ctrl Pts',(23.5690408995974,9.24743420487348,-0.0682698870437648));
#30183=CARTESIAN_POINT('Ctrl Pts',(23.5690458054721,9.24743408929769,-0.0682706755863066));
#30184=CARTESIAN_POINT('Ctrl Pts',(23.5690507113481,9.24743397371795,-0.0682714641170214));
#30185=CARTESIAN_POINT('Ctrl Pts',(23.6442548651033,9.24566220524802,-0.0803591696110631));
#30186=CARTESIAN_POINT('Ctrl Pts',(23.719780223829,9.24296231063544,-0.0896678135679566));
#30187=CARTESIAN_POINT('Ctrl Pts',(23.7952824304768,9.23933323520794,-0.098112337331162));
#30188=CARTESIAN_POINT('Ctrl Pts',(23.795287196916,9.23933300610514,-0.0981128704322552));
#30189=CARTESIAN_POINT('Ctrl Pts',(23.7952919633553,9.23933277699862,-0.0981134035295249));
#30190=CARTESIAN_POINT('Ctrl Pts',(23.7952967297948,9.23933254788841,-0.0981139366229708));
#30191=CARTESIAN_POINT('Ctrl Pts',(23.9463062361403,9.23207391784971,-0.115003310510118));
#30192=CARTESIAN_POINT('Ctrl Pts',(24.0974556990499,9.22109573441987,-0.128054897542612));
#30193=CARTESIAN_POINT('Ctrl Pts',(24.2484785175586,9.20637641464955,-0.139900632118544));
#30194=CARTESIAN_POINT('Ctrl Pts',(24.2484829666272,9.2063759810246,-0.139900981088888));
#30195=CARTESIAN_POINT('Ctrl Pts',(24.2484874156951,9.20637554739644,-0.139901330058036));
#30196=CARTESIAN_POINT('Ctrl Pts',(24.2484918647625,9.20637511376508,-0.139901679025988));
#30197=CARTESIAN_POINT('Ctrl Pts',(24.5505425107233,9.17693554307987,-0.163593384587027));
#30198=CARTESIAN_POINT('Ctrl Pts',(24.8500228881277,9.13271031628177,-0.181771961304202));
#30199=CARTESIAN_POINT('Ctrl Pts',(25.1449954475175,9.07440073882145,-0.198110501056529));
#30200=CARTESIAN_POINT('Ctrl Pts',(25.1449991716412,9.07440000264425,-0.19811070733586));
#30201=CARTESIAN_POINT('Ctrl Pts',(25.1450028957642,9.0743992664648,-0.198110913614874));
#30202=CARTESIAN_POINT('Ctrl Pts',(25.1450066198866,9.07439853028311,-0.198111119893571));
#30203=CARTESIAN_POINT('Ctrl Pts',(25.734956508507,8.95777768468516,-0.23078837411552));
#30204=CARTESIAN_POINT('Ctrl Pts',(26.3094088549805,8.78499087735302,-0.255519529851774));
#30205=CARTESIAN_POINT('Ctrl Pts',(26.8679234097883,8.55541116229534,-0.27759745040406));
#30206=CARTESIAN_POINT('Ctrl Pts',(26.867925760244,8.5554101961308,-0.277597543316903));
#30207=CARTESIAN_POINT('Ctrl Pts',(26.8679281106996,8.55540922996518,-0.277597636229693));
#30208=CARTESIAN_POINT('Ctrl Pts',(26.8679304611549,8.5554082637985,-0.277597729142428));
#30209=CARTESIAN_POINT('Ctrl Pts',(27.1471871052162,8.44061839374216,-0.288636653344279));
#30210=CARTESIAN_POINT('Ctrl Pts',(27.4237272806306,8.31073561236966,-0.298912461553731));
#30211=CARTESIAN_POINT('Ctrl Pts',(27.6907408700783,8.16889014503095,-0.308412822043665));
#30212=CARTESIAN_POINT('Ctrl Pts',(27.6907425556339,8.16888924961423,-0.308412882015843));
#30213=CARTESIAN_POINT('Ctrl Pts',(27.6907442411893,8.16888835419702,-0.308412941987992));
#30214=CARTESIAN_POINT('Ctrl Pts',(27.6907459267443,8.16888745877932,-0.308413001960112));
#30215=CARTESIAN_POINT('Ctrl Pts',(27.9577599700424,8.02704153892829,-0.317913373144742));
#30216=CARTESIAN_POINT('Ctrl Pts',(28.2162196174067,7.8729946215703,-0.326677439449265));
#30217=CARTESIAN_POINT('Ctrl Pts',(28.4663064740913,7.7070127601481,-0.334872469822339));
#30218=CARTESIAN_POINT('Ctrl Pts',(28.4663075265582,7.70701206162913,-0.33487250431035));
#30219=CARTESIAN_POINT('Ctrl Pts',(28.4663085790249,7.70701136310996,-0.33487253879835));
#30220=CARTESIAN_POINT('Ctrl Pts',(28.4663096314915,7.70701066459057,-0.33487257328634));
#30221=CARTESIAN_POINT('Ctrl Pts',(28.9070555201026,7.4144887448157,-0.34931525499634));
#30222=CARTESIAN_POINT('Ctrl Pts',(29.3219854583099,7.08516810894049,-0.362013648044849));
#30223=CARTESIAN_POINT('Ctrl Pts',(29.7101085977472,6.71766015929422,-0.373413798110151));
#30224=CARTESIAN_POINT('Ctrl Pts',(29.7624427821908,6.66810570899995,-0.374950984367759));
#30225=CARTESIAN_POINT('Ctrl Pts',(29.8142895317361,6.6178568890955,-0.376464564268085));
#30226=CARTESIAN_POINT('Ctrl Pts',(29.8656463748334,6.56691023510737,-0.377955629499264));
#30227=CARTESIAN_POINT('',(23.3621597248275,-9.24999241530675,-0.0116776286864305));
#30228=CARTESIAN_POINT('Ctrl Pts',(29.8656463748335,-6.5669102351073,-0.377955629499294));
#30229=CARTESIAN_POINT('Ctrl Pts',(29.4847714407085,-6.94474310627589,-0.366897524338192));
#30230=CARTESIAN_POINT('Ctrl Pts',(29.0769538041632,-7.28419815787297,-0.354601205857789));
#30231=CARTESIAN_POINT('Ctrl Pts',(28.6431883543724,-7.58666973512015,-0.340620835122163));
#30232=CARTESIAN_POINT('Ctrl Pts',(28.5846997977317,-7.62745473998063,-0.338735734070377));
#30233=CARTESIAN_POINT('Ctrl Pts',(28.5257394240778,-7.66756726314656,-0.336820011942593));
#30234=CARTESIAN_POINT('Ctrl Pts',(28.4663096314912,-7.70701066459059,-0.334872573291177));
#30235=CARTESIAN_POINT('Ctrl Pts',(28.4663085790239,-7.70701136311043,-0.334872538803164));
#30236=CARTESIAN_POINT('Ctrl Pts',(28.4663075265564,-7.70701206163006,-0.334872504315141));
#30237=CARTESIAN_POINT('Ctrl Pts',(28.4663064740889,-7.70701276014948,-0.334872469827109));
#30238=CARTESIAN_POINT('Ctrl Pts',(28.2162196174051,-7.87299462157124,-0.326677439449156));
#30239=CARTESIAN_POINT('Ctrl Pts',(27.9577599700418,-8.02704153892891,-0.317913373136687));
#30240=CARTESIAN_POINT('Ctrl Pts',(27.6907459267442,-8.1688874587795,-0.308413001956161));
#30241=CARTESIAN_POINT('Ctrl Pts',(27.6907442411881,-8.16888835419778,-0.308412941984002));
#30242=CARTESIAN_POINT('Ctrl Pts',(27.6907425556317,-8.16888924961559,-0.308412882011813));
#30243=CARTESIAN_POINT('Ctrl Pts',(27.6907408700749,-8.16889014503291,-0.308412822039595));
#30244=CARTESIAN_POINT('Ctrl Pts',(27.4237272806281,-8.31073561237086,-0.298912461553772));
#30245=CARTESIAN_POINT('Ctrl Pts',(27.1471871052143,-8.44061839374265,-0.288636653353161));
#30246=CARTESIAN_POINT('Ctrl Pts',(26.8679304611544,-8.55540826379855,-0.277597729148227));
#30247=CARTESIAN_POINT('Ctrl Pts',(26.8679281106974,-8.55540922996587,-0.27759763623543));
#30248=CARTESIAN_POINT('Ctrl Pts',(26.8679257602403,-8.55541019613213,-0.277597543322579));
#30249=CARTESIAN_POINT('Ctrl Pts',(26.867923409783,-8.55541116229733,-0.277597450409673));
#30250=CARTESIAN_POINT('Ctrl Pts',(26.309408854977,-8.78499087735412,-0.255519529851172));
#30251=CARTESIAN_POINT('Ctrl Pts',(25.7349565085049,-8.9577776846856,-0.23078837411658));
#30252=CARTESIAN_POINT('Ctrl Pts',(25.1450066198861,-9.07439853028321,-0.198111119893957));
#30253=CARTESIAN_POINT('Ctrl Pts',(25.1450028957612,-9.07439926646539,-0.198110913615121));
#30254=CARTESIAN_POINT('Ctrl Pts',(25.1449991716356,-9.07440000264534,-0.198110707335968));
#30255=CARTESIAN_POINT('Ctrl Pts',(25.1449954475095,-9.07440073882304,-0.198110501056499));
#30256=CARTESIAN_POINT('Ctrl Pts',(24.8500228881221,-9.13271031628261,-0.181771961303894));
#30257=CARTESIAN_POINT('Ctrl Pts',(24.5505425107174,-9.1769355430799,-0.163593384622763));
#30258=CARTESIAN_POINT('Ctrl Pts',(24.2484918647611,-9.20637511376504,-0.139901679037309));
#30259=CARTESIAN_POINT('Ctrl Pts',(24.2484874156906,-9.20637554739671,-0.139901330069121));
#30260=CARTESIAN_POINT('Ctrl Pts',(24.2484829666197,-9.20637598102516,-0.139900981099737));
#30261=CARTESIAN_POINT('Ctrl Pts',(24.2484785175481,-9.2063764146504,-0.139900632129157));
#30262=CARTESIAN_POINT('Ctrl Pts',(24.0974556990432,-9.22109573442037,-0.128054897541096));
#30263=CARTESIAN_POINT('Ctrl Pts',(23.9463062361367,-9.2320739178499,-0.115003310509656));
#30264=CARTESIAN_POINT('Ctrl Pts',(23.7952967297941,-9.23933254788843,-0.0981139366229608));
#30265=CARTESIAN_POINT('Ctrl Pts',(23.7952919633514,-9.23933277699881,-0.0981134035291551));
#30266=CARTESIAN_POINT('Ctrl Pts',(23.7952871969089,-9.23933300610547,-0.0981128704315258));
#30267=CARTESIAN_POINT('Ctrl Pts',(23.7952824304665,-9.23933323520843,-0.0981123373300727));
#30268=CARTESIAN_POINT('Ctrl Pts',(23.7197802238219,-9.2429623106357,-0.0896678135672034));
#30269=CARTESIAN_POINT('Ctrl Pts',(23.6442548650996,-9.24566220524811,-0.0803591696095396));
#30270=CARTESIAN_POINT('Ctrl Pts',(23.5690507113475,-9.24743397371796,-0.068271464116656));
#30271=CARTESIAN_POINT('Ctrl Pts',(23.5690458054681,-9.24743408929778,-0.0682706755854086));
#30272=CARTESIAN_POINT('Ctrl Pts',(23.5690408995901,-9.24743420487365,-0.068269887042334));
#30273=CARTESIAN_POINT('Ctrl Pts',(23.5690359937135,-9.24743432044557,-0.0682690984874317));
#30274=CARTESIAN_POINT('Ctrl Pts',(23.5314364698732,-9.24832008448463,-0.0622254714293397));
#30275=CARTESIAN_POINT('Ctrl Pts',(23.4939660705731,-9.24897214983,-0.055571723955567));
#30276=CARTESIAN_POINT('Ctrl Pts',(23.4569292913262,-9.2493955706006,-0.0469072991570471));
#30277=CARTESIAN_POINT('Ctrl Pts',(23.4569243811925,-9.24939562673541,-0.0469061504749738));
#30278=CARTESIAN_POINT('Ctrl Pts',(23.4569194710664,-9.2493956828662,-0.0469050017575602));
#30279=CARTESIAN_POINT('Ctrl Pts',(23.4569145609479,-9.24939573899298,-0.0469038530048031));
#30280=CARTESIAN_POINT('Ctrl Pts',(23.4383987227168,-9.24960739055848,-0.0425719574877666));
#30281=CARTESIAN_POINT('Ctrl Pts',(23.4199770709982,-9.24976189104565,-0.0378028340633931));
#30282=CARTESIAN_POINT('Ctrl Pts',(23.4018877334049,-9.24986104529552,-0.0315011520350705));
#30283=CARTESIAN_POINT('Ctrl Pts',(23.4018828933734,-9.2498610718255,-0.0314994659402038));
#30284=CARTESIAN_POINT('Ctrl Pts',(23.4018780533658,-9.24986109835151,-0.0314977797355663));
#30285=CARTESIAN_POINT('Ctrl Pts',(23.4018732133819,-9.24986112487356,-0.031496093421139));
#30286=CARTESIAN_POINT('Ctrl Pts',(23.3928310750493,-9.24991067381161,-0.0283456927611094));
#30287=CARTESIAN_POINT('Ctrl Pts',(23.3838350766164,-9.24994620152362,-0.0248366031008535));
#30288=CARTESIAN_POINT('Ctrl Pts',(23.3754258633825,-9.24996824007847,-0.0202870718871724));
#30289=CARTESIAN_POINT('Ctrl Pts',(23.3754221035648,-9.24996824993206,-0.0202850377600923));
#30290=CARTESIAN_POINT('Ctrl Pts',(23.3754183438643,-9.24996825978296,-0.0202830034249692));
#30291=CARTESIAN_POINT('Ctrl Pts',(23.3754145842812,-9.24996826963115,-0.0202809688817427));
#30292=CARTESIAN_POINT('Ctrl Pts',(23.3709568489949,-9.24997994663257,-0.0178686122552752));
#30293=CARTESIAN_POINT('Ctrl Pts',(23.3659604527863,-9.249987704137,-0.0151874246645509));
#30294=CARTESIAN_POINT('Ctrl Pts',(23.3621597248275,-9.24999241530675,-0.0116776286864305));
#30295=CARTESIAN_POINT('',(23.3621596556826,-5.66399144605651E-16,9.25));
#30296=CARTESIAN_POINT('Origin',(23.3621596556826,0.,0.));
#30297=CARTESIAN_POINT('',(23.3560798393748,-9.24999818736112,-1.077153489017E-8));
#30298=CARTESIAN_POINT('Ctrl Pts',(23.3621597248275,-9.24999241530675,-0.0116776286864305));
#30299=CARTESIAN_POINT('Ctrl Pts',(23.3587904572015,-9.24999659166241,-0.00856626631297116));
#30300=CARTESIAN_POINT('Ctrl Pts',(23.3563609263675,-9.24999837416356,-0.00480370845307387));
#30301=CARTESIAN_POINT('Ctrl Pts',(23.3560798285161,-9.24999837277875,-1.1406897794386E-8));
#30302=CARTESIAN_POINT('',(16.3220957355182,-6.,0.));
#30303=CARTESIAN_POINT('Origin',(23.3621596556826,0.,0.));
#30304=CARTESIAN_POINT('',(16.3220957355182,6.,0.));
#30305=CARTESIAN_POINT('Origin',(16.3220957355182,0.,0.));
#30306=CARTESIAN_POINT('Origin',(23.3621596556826,0.,0.));
#30307=CARTESIAN_POINT('Origin',(23.3621596556826,0.,0.));
#30308=CARTESIAN_POINT('',(12.9815732451447,2.54439044914164E-11,-11.0119484097524));
#30309=CARTESIAN_POINT('',(23.3608103941008,-11.1532440216953,-5.06593335958171));
#30310=CARTESIAN_POINT('Ctrl Pts',(12.9815732451008,2.5445788709682E-11,
-11.0119484101204));
#30311=CARTESIAN_POINT('Ctrl Pts',(12.9815732274295,-0.383296294064764,
-11.0119485582815));
#30312=CARTESIAN_POINT('Ctrl Pts',(12.9993217484721,-0.765312998797785,
-10.9941006207665));
#30313=CARTESIAN_POINT('Ctrl Pts',(13.0347559988626,-1.1460555907501,-10.9585267749209));
#30314=CARTESIAN_POINT('Ctrl Pts',(13.0368286609663,-1.16832643697724,-10.9564459474346));
#30315=CARTESIAN_POINT('Ctrl Pts',(13.0389618718051,-1.19059290057529,-10.9543044712817));
#30316=CARTESIAN_POINT('Ctrl Pts',(13.0411556343664,-1.21285503798338,-10.9521023639809));
#30317=CARTESIAN_POINT('Ctrl Pts',(13.0673836657568,-1.47901512706784,-10.9257745651442));
#30318=CARTESIAN_POINT('Ctrl Pts',(13.1025879418344,-1.74579707980255,-10.8904589178109));
#30319=CARTESIAN_POINT('Ctrl Pts',(13.1460558221011,-2.00934344707994,-10.8469554421057));
#30320=CARTESIAN_POINT('Ctrl Pts',(13.1611087883244,-2.10060979226513,-10.83189014915));
#30321=CARTESIAN_POINT('Ctrl Pts',(13.1771529803443,-2.19148779862728,-10.81584273198));
#30322=CARTESIAN_POINT('Ctrl Pts',(13.1941594450425,-2.28181600059225,-10.798845827919));
#30323=CARTESIAN_POINT('Ctrl Pts',(13.2023910039891,-2.32553713442028,-10.7906188965626));
#30324=CARTESIAN_POINT('Ctrl Pts',(13.2108484018431,-2.36913426878318,-10.7821685435845));
#30325=CARTESIAN_POINT('Ctrl Pts',(13.2195283907449,-2.4125885817506,-10.7734983679309));
#30326=CARTESIAN_POINT('Ctrl Pts',(13.3201001314545,-2.91607723201734,-10.6730403296062));
#30327=CARTESIAN_POINT('Ctrl Pts',(13.4501508634135,-3.4036814155668,-10.5433923350781));
#30328=CARTESIAN_POINT('Ctrl Pts',(13.6081630039645,-3.87613361463931,-10.3871346982887));
#30329=CARTESIAN_POINT('Ctrl Pts',(13.6691942514409,-4.05861546053914,-10.3267811174328));
#30330=CARTESIAN_POINT('Ctrl Pts',(13.7343973267524,-4.23883645844413,-10.2624577747158));
#30331=CARTESIAN_POINT('Ctrl Pts',(13.8036860977875,-4.41683730799235,-10.1943136878064));
#30332=CARTESIAN_POINT('Ctrl Pts',(13.8328199711978,-4.49168138647981,-10.1656611201245));
#30333=CARTESIAN_POINT('Ctrl Pts',(13.8626775326182,-4.56611464018205,-10.1363412173927));
#30334=CARTESIAN_POINT('Ctrl Pts',(13.8932514259218,-4.64014509869768,-10.1063639362644));
#30335=CARTESIAN_POINT('Ctrl Pts',(13.9943512020743,-4.88494423860655,-10.0072369987289));
#30336=CARTESIAN_POINT('Ctrl Pts',(14.1019598843113,-5.1222638353909,-9.90221549601681));
#30337=CARTESIAN_POINT('Ctrl Pts',(14.2158396515836,-5.35278002273372,-9.79173341205274));
#30338=CARTESIAN_POINT('Ctrl Pts',(14.2236525199707,-5.36859488323034,-9.78415364611349));
#30339=CARTESIAN_POINT('Ctrl Pts',(14.2314949176702,-5.38437771263948,-9.77654816486061));
#30340=CARTESIAN_POINT('Ctrl Pts',(14.2393667732968,-5.40012872553306,-9.76891710267621));
#30341=CARTESIAN_POINT('Ctrl Pts',(14.3650579854142,-5.65162773625904,-9.64707067901238));
#30342=CARTESIAN_POINT('Ctrl Pts',(14.4981847686049,-5.89496716334364,-9.51871404350092));
#30343=CARTESIAN_POINT('Ctrl Pts',(14.6384789849032,-6.13072391768223,-9.38459915056585));
#30344=CARTESIAN_POINT('Ctrl Pts',(14.6737714708389,-6.19003100928071,-9.35086113842561));
#30345=CARTESIAN_POINT('Ctrl Pts',(14.7095174354231,-6.24885832423709,-9.31675895403165));
#30346=CARTESIAN_POINT('Ctrl Pts',(14.7457124150901,-6.30721521168454,-9.28230502718912));
#30347=CARTESIAN_POINT('Ctrl Pts',(14.7998381789771,-6.39448176467667,-9.23078282365662));
#30348=CARTESIAN_POINT('Ctrl Pts',(14.8549715128261,-6.48069604666143,-9.17847475902765));
#30349=CARTESIAN_POINT('Ctrl Pts',(14.9110921849357,-6.56589391149648,-9.12541926115511));
#30350=CARTESIAN_POINT('Ctrl Pts',(15.041685362699,-6.76414991038648,-9.00195876425546));
#30351=CARTESIAN_POINT('Ctrl Pts',(15.1776986530004,-6.95682139014027,-8.87440061067004));
#30352=CARTESIAN_POINT('Ctrl Pts',(15.3191490883084,-7.1441213175117,-8.74313806886841));
#30353=CARTESIAN_POINT('Ctrl Pts',(15.386104712241,-7.2327798180839,-8.68100488867582));
#30354=CARTESIAN_POINT('Ctrl Pts',(15.4543283803757,-7.32029479475722,-8.61799959364879));
#30355=CARTESIAN_POINT('Ctrl Pts',(15.5237866306372,-7.40663268301795,-8.55420191705971));
#30356=CARTESIAN_POINT('Ctrl Pts',(15.631823395544,-7.54092437769016,-8.45496972273705));
#30357=CARTESIAN_POINT('Ctrl Pts',(15.7425934164994,-7.67199804493825,-8.35406036021674));
#30358=CARTESIAN_POINT('Ctrl Pts',(15.8555749280103,-7.79941820934665,-8.25217221569744));
#30359=CARTESIAN_POINT('Ctrl Pts',(15.8893542526762,-7.83751441681426,-8.22170959692655));
#30360=CARTESIAN_POINT('Ctrl Pts',(15.9233310534103,-7.87528429890062,-8.19115961757327));
#30361=CARTESIAN_POINT('Ctrl Pts',(15.9574908972915,-7.91271690993404,-8.16054121449193));
#30362=CARTESIAN_POINT('Ctrl Pts',(16.0364328953598,-7.99922213865137,-8.08978334085214));
#30363=CARTESIAN_POINT('Ctrl Pts',(16.1164661586433,-8.0840494038951,-8.01855942060974));
#30364=CARTESIAN_POINT('Ctrl Pts',(16.1974689739095,-8.167105566649,-7.94705648567565));
#30365=CARTESIAN_POINT('Ctrl Pts',(16.3862511497973,-8.36067319851518,-7.78041438077027));
#30366=CARTESIAN_POINT('Ctrl Pts',(16.5808510409098,-8.54531969831238,-7.6117230894063));
#30367=CARTESIAN_POINT('Ctrl Pts',(16.7815955192347,-8.72152156029507,-7.44211131482556));
#30368=CARTESIAN_POINT('Ctrl Pts',(16.8274598051923,-8.76177857085733,-7.40335994793335));
#30369=CARTESIAN_POINT('Ctrl Pts',(16.8736448373626,-8.80159493353399,-7.36456068417118));
#30370=CARTESIAN_POINT('Ctrl Pts',(16.9201545218898,-8.84097660013473,-7.32572724718514));
#30371=CARTESIAN_POINT('Ctrl Pts',(17.073716166418,-8.97100357298887,-7.19751037134778));
#30372=CARTESIAN_POINT('Ctrl Pts',(17.2308071180094,-9.09628923719283,-7.06890359935271));
#30373=CARTESIAN_POINT('Ctrl Pts',(17.3917693612564,-9.21694196463097,-6.94059501703444));
#30374=CARTESIAN_POINT('Ctrl Pts',(17.4912340889155,-9.29149790044471,-6.8613082356181));
#30375=CARTESIAN_POINT('Ctrl Pts',(17.5922012020707,-9.3642909638437,-6.78213270267914));
#30376=CARTESIAN_POINT('Ctrl Pts',(17.6947656292074,-9.43536158302822,-6.70321570188847));
#30377=CARTESIAN_POINT('Ctrl Pts',(17.8575457281888,-9.54815782972409,-6.5779664555498));
#30378=CARTESIAN_POINT('Ctrl Pts',(18.0243246162118,-9.65661829996039,-6.45333491604299));
#30379=CARTESIAN_POINT('Ctrl Pts',(18.1958339964268,-9.76078864798243,-6.33031238527626));
#30380=CARTESIAN_POINT('Ctrl Pts',(18.3051389765451,-9.82717765717364,-6.25190865445575));
#30381=CARTESIAN_POINT('Ctrl Pts',(18.416470201457,-9.89187030973724,-6.17410893862717));
#30382=CARTESIAN_POINT('Ctrl Pts',(18.5299490632647,-9.95482201107074,-6.09724150236054));
#30383=CARTESIAN_POINT('Ctrl Pts',(18.6919068330151,-10.0446670887139,-5.98753579729915));
#30384=CARTESIAN_POINT('Ctrl Pts',(18.8582821726837,-10.1309242043064,-5.87972874713949));
#30385=CARTESIAN_POINT('Ctrl Pts',(19.028597750893,-10.2129461794984,-5.77597483478962));
#30386=CARTESIAN_POINT('Ctrl Pts',(19.0441752064857,-10.220448098522,-5.76648526267183));
#30387=CARTESIAN_POINT('Ctrl Pts',(19.0597855949024,-10.2279146095031,-5.75702960254959));
#30388=CARTESIAN_POINT('Ctrl Pts',(19.0754285341388,-10.2353452303139,-5.74760950379945));
#30389=CARTESIAN_POINT('Ctrl Pts',(19.1939081940033,-10.2916247704269,-5.6762616529295));
#30390=CARTESIAN_POINT('Ctrl Pts',(19.3144152371265,-10.3459177594171,-5.6068633280272));
#30391=CARTESIAN_POINT('Ctrl Pts',(19.4368829990435,-10.3980330380265,-5.54011236932002));
#30392=CARTESIAN_POINT('Ctrl Pts',(19.5831223220011,-10.4602641341148,-5.46040473969324));
#30393=CARTESIAN_POINT('Ctrl Pts',(19.7324596468288,-10.5195440088144,-5.38432247817642));
#30394=CARTESIAN_POINT('Ctrl Pts',(19.8855045724414,-10.5757459074742,-5.31311389279469));
#30395=CARTESIAN_POINT('Ctrl Pts',(19.8962358389881,-10.5796866951386,-5.30812086014703));
#30396=CARTESIAN_POINT('Ctrl Pts',(19.9069853432655,-10.5836123466384,-5.30315180853967));
#30397=CARTESIAN_POINT('Ctrl Pts',(19.9177532995298,-10.5875228169023,-5.29820717709418));
#30398=CARTESIAN_POINT('Ctrl Pts',(19.9575183005516,-10.6019637981082,-5.27994714058804));
#30399=CARTESIAN_POINT('Ctrl Pts',(19.9975491622602,-10.6162022971217,-5.26201449196818));
#30400=CARTESIAN_POINT('Ctrl Pts',(20.0378492890609,-10.6302309693699,-5.24444185690922));
#30401=CARTESIAN_POINT('Ctrl Pts',(20.1630026639133,-10.6737974743894,-5.18986945832715));
#30402=CARTESIAN_POINT('Ctrl Pts',(20.2908483914919,-10.7153750760828,-5.13872259572955));
#30403=CARTESIAN_POINT('Ctrl Pts',(20.4214038079289,-10.754702500542,-5.0920472070559));
#30404=CARTESIAN_POINT('Ctrl Pts',(20.5928781972893,-10.8063560150289,-5.03074271284645));
#30405=CARTESIAN_POINT('Ctrl Pts',(20.7671691077214,-10.8535702841615,-4.9778372816226));
#30406=CARTESIAN_POINT('Ctrl Pts',(20.94442935131,-10.8960769893133,-4.93523064039145));
#30407=CARTESIAN_POINT('Ctrl Pts',(20.995814496353,-10.9083990597636,-4.9228795999374));
#30408=CARTESIAN_POINT('Ctrl Pts',(21.0474492395618,-10.9203258484385,-4.91139488931843));
#30409=CARTESIAN_POINT('Ctrl Pts',(21.09933747016,-10.9318487261951,-4.90082131360441));
#30410=CARTESIAN_POINT('Ctrl Pts',(21.2255805168313,-10.9598836616254,-4.87509601141239));
#30411=CARTESIAN_POINT('Ctrl Pts',(21.353441387833,-10.9855508187274,-4.85474602453125));
#30412=CARTESIAN_POINT('Ctrl Pts',(21.4828826861467,-11.0087074356192,-4.84043539750503));
#30413=CARTESIAN_POINT('Ctrl Pts',(21.5416752221987,-11.0192252243867,-4.83393547772421));
#30414=CARTESIAN_POINT('Ctrl Pts',(21.6009563602522,-11.0292416622094,-4.8286938697609));
#30415=CARTESIAN_POINT('Ctrl Pts',(21.6605166873071,-11.0387197298414,-4.82474839119763));
#30416=CARTESIAN_POINT('Ctrl Pts',(21.7393049199761,-11.0512576092448,-4.81952919079354));
#30417=CARTESIAN_POINT('Ctrl Pts',(21.8188480608857,-11.0628933590837,-4.81656587560977));
#30418=CARTESIAN_POINT('Ctrl Pts',(21.8984893540544,-11.0735048808963,-4.81597836766281));
#30419=CARTESIAN_POINT('Ctrl Pts',(21.9447446265687,-11.0796680007266,-4.81563714592834));
#30420=CARTESIAN_POINT('Ctrl Pts',(21.9910325842705,-11.0854859487789,-4.81609650321322));
#30421=CARTESIAN_POINT('Ctrl Pts',(22.0372232100108,-11.0909378851566,-4.81737257485754));
#30422=CARTESIAN_POINT('Ctrl Pts',(22.1039899135981,-11.0988184413143,-4.81921708542365));
#30423=CARTESIAN_POINT('Ctrl Pts',(22.1705282673233,-11.1059466127202,-4.82273204984088));
#30424=CARTESIAN_POINT('Ctrl Pts',(22.2367244241683,-11.1123321983582,-4.82784959532291));
#30425=CARTESIAN_POINT('Ctrl Pts',(22.3548448203634,-11.1237266348551,-4.8369813414649));
#30426=CARTESIAN_POINT('Ctrl Pts',(22.47218105154,-11.1327897089269,-4.85123108401182));
#30427=CARTESIAN_POINT('Ctrl Pts',(22.5888357694595,-11.139637195494,-4.87030011174849));
#30428=CARTESIAN_POINT('Ctrl Pts',(22.7297473141248,-11.1479085275624,-4.89333429503368));
#30429=CARTESIAN_POINT('Ctrl Pts',(22.8696658790769,-11.1529476864071,-4.9233902362237));
#30430=CARTESIAN_POINT('Ctrl Pts',(23.0087902947259,-11.1548965106162,-4.95984270507666));
#30431=CARTESIAN_POINT('Ctrl Pts',(23.0499434250456,-11.1554729746126,-4.9706253789458));
#30432=CARTESIAN_POINT('Ctrl Pts',(23.0910270302596,-11.1557788974522,-4.98196805853579));
#30433=CARTESIAN_POINT('Ctrl Pts',(23.1320461648849,-11.1558175993799,-4.99385533031318));
#30434=CARTESIAN_POINT('Ctrl Pts',(23.2085117001587,-11.15588974531,-5.01601490553846));
#30435=CARTESIAN_POINT('Ctrl Pts',(23.2848869024912,-11.1550160733614,-5.04013662844268));
#30436=CARTESIAN_POINT('Ctrl Pts',(23.3608104906557,-11.1532443098673,-5.06593275297875));
#30437=CARTESIAN_POINT('',(23.3622216893479,-11.1611076779314,-5.04898962599655));
#30438=CARTESIAN_POINT('Ctrl Pts',(23.3609338235094,-11.1532508593964,-5.06595631491688));
#30439=CARTESIAN_POINT('Ctrl Pts',(23.3613828231202,-11.1545850969447,-5.06314833543963));
#30440=CARTESIAN_POINT('Ctrl Pts',(23.3617214043993,-11.1559114660996,-5.06032297389091));
#30441=CARTESIAN_POINT('Ctrl Pts',(23.3621711199265,-11.1585366545092,-5.05466150053041));
#30442=CARTESIAN_POINT('Ctrl Pts',(23.3622835506299,-11.1598325219751,-5.05183232221884));
#30443=CARTESIAN_POINT('Ctrl Pts',(23.3622837237339,-11.161116664397,-5.04899369509034));
#30444=CARTESIAN_POINT('',(23.3621596556826,-1.50019232895551E-15,12.25));
#30445=CARTESIAN_POINT('Origin',(23.3621596556826,0.,0.));
#30446=CARTESIAN_POINT('',(23.3621596556826,-1.50019232895551E-15,12.25));
#30447=CARTESIAN_POINT('',(23.3621596556826,11.1611032572144,-5.04898743133702));
#30448=CARTESIAN_POINT('Origin',(23.3621596556826,0.,0.));
#30449=CARTESIAN_POINT('',(23.3608199268969,11.1532686296421,-5.06590764537049));
#30450=CARTESIAN_POINT('Origin',(23.2960504456339,11.1496971587182,-5.05333275681839));
#30451=CARTESIAN_POINT('Ctrl Pts',(23.3608199267208,11.1532599621143,-5.06590352720005));
#30452=CARTESIAN_POINT('Ctrl Pts',(23.2851099168874,11.1550241480784,-5.04018501841967));
#30453=CARTESIAN_POINT('Ctrl Pts',(23.2088153626835,11.1558905993071,-5.01610178142038));
#30454=CARTESIAN_POINT('Ctrl Pts',(23.1319091372516,11.1558170356561,-4.99381659031829));
#30455=CARTESIAN_POINT('Ctrl Pts',(23.0065821941946,11.1556971557966,-4.95750048117918));
#30456=CARTESIAN_POINT('Ctrl Pts',(22.8810022185292,11.1530840174098,-4.92636875508836));
#30457=CARTESIAN_POINT('Ctrl Pts',(22.7549925111962,11.1479188168036,-4.90077017644917));
#30458=CARTESIAN_POINT('Ctrl Pts',(22.6986428750304,11.1456090171775,-4.88932287906862));
#30459=CARTESIAN_POINT('Ctrl Pts',(22.6422072591868,11.142788578058,-4.87898266372752));
#30460=CARTESIAN_POINT('Ctrl Pts',(22.5856696257093,11.1394507867115,-4.86978382109285));
#30461=CARTESIAN_POINT('Ctrl Pts',(22.4680192465019,11.1325051048096,-4.85064175133027));
#30462=CARTESIAN_POINT('Ctrl Pts',(22.3499266942736,11.1233201691922,-4.83644525304962));
#30463=CARTESIAN_POINT('Ctrl Pts',(22.2312576655186,11.1118030090012,-4.82743144527622));
#30464=CARTESIAN_POINT('Ctrl Pts',(22.1656422229571,11.1054348473088,-4.8224474575212));
#30465=CARTESIAN_POINT('Ctrl Pts',(22.0998654322016,11.0983545374085,-4.81905040982186));
#30466=CARTESIAN_POINT('Ctrl Pts',(22.0339388739251,11.0905496356051,-4.81728321117063));
#30467=CARTESIAN_POINT('Ctrl Pts',(21.9082231125919,11.0756664201302,-4.81391332914321));
#30468=CARTESIAN_POINT('Ctrl Pts',(21.7814080631358,11.0580224086786,-4.81659458033227));
#30469=CARTESIAN_POINT('Ctrl Pts',(21.655559184383,11.0379275898652,-4.82508454412653));
#30470=CARTESIAN_POINT('Ctrl Pts',(21.5963315189804,11.0284704598788,-4.82908013582245));
#30471=CARTESIAN_POINT('Ctrl Pts',(21.5373996159708,11.0184845836996,-4.83435441281115));
#30472=CARTESIAN_POINT('Ctrl Pts',(21.4789497009406,11.0080025426114,-4.84087311309483));
#30473=CARTESIAN_POINT('Ctrl Pts',(21.3622279367936,10.9870703936589,-4.85389065463726));
#30474=CARTESIAN_POINT('Ctrl Pts',(21.2470582382663,10.9641488738826,-4.87177728137055));
#30475=CARTESIAN_POINT('Ctrl Pts',(21.1332169561902,10.939307337495,-4.89405377843275));
#30476=CARTESIAN_POINT('Ctrl Pts',(21.1194119170954,10.9362949119956,-4.89675515272537));
#30477=CARTESIAN_POINT('Ctrl Pts',(21.1056264289217,10.9332542308073,-4.89952113826779));
#30478=CARTESIAN_POINT('Ctrl Pts',(21.0918601058164,10.9301854003157,-4.90235092599176));
#30479=CARTESIAN_POINT('Ctrl Pts',(21.0405875008949,10.9187555557478,-4.91289045690887));
#30480=CARTESIAN_POINT('Ctrl Pts',(20.9895925706238,10.9069380473771,-4.92431218409081));
#30481=CARTESIAN_POINT('Ctrl Pts',(20.9388639538911,10.8947409567297,-4.93657125545549));
#30482=CARTESIAN_POINT('Ctrl Pts',(20.8074102624665,10.8631344850081,-4.96833833857571));
#30483=CARTESIAN_POINT('Ctrl Pts',(20.6777434435588,10.8289788908431,-5.00571952389078));
#30484=CARTESIAN_POINT('Ctrl Pts',(20.5496792463686,10.7923623174254,-5.04795262161033));
#30485=CARTESIAN_POINT('Ctrl Pts',(20.5047265821631,10.779509290855,-5.06277714166981));
#30486=CARTESIAN_POINT('Ctrl Pts',(20.4599587538759,10.766349077854,-5.07820447630388));
#30487=CARTESIAN_POINT('Ctrl Pts',(20.4153833864829,10.7528895773077,-5.09419756001321));
#30488=CARTESIAN_POINT('Ctrl Pts',(20.2991843165291,10.7178033506092,-5.13588833142814));
#30489=CARTESIAN_POINT('Ctrl Pts',(20.1850131651627,10.6808901991499,-5.18117061724925));
#30490=CARTESIAN_POINT('Ctrl Pts',(20.0732309971985,10.6424705764709,-5.22913387074176));
#30491=CARTESIAN_POINT('Ctrl Pts',(20.0585888700092,10.637438065364,-5.23541648335201));
#30492=CARTESIAN_POINT('Ctrl Pts',(20.0439876792257,10.6323797376686,-5.24174505771744));
#30493=CARTESIAN_POINT('Ctrl Pts',(20.0294281869367,10.6272963400987,-5.24811751925262));
#30494=CARTESIAN_POINT('Ctrl Pts',(19.9899973548944,10.6135291982364,-5.26537577630607));
#30495=CARTESIAN_POINT('Ctrl Pts',(19.9508410932218,10.5995670286226,-5.28297007979696));
#30496=CARTESIAN_POINT('Ctrl Pts',(19.9119646421441,10.5854198612558,-5.30086579628549));
#30497=CARTESIAN_POINT('Ctrl Pts',(19.7480083757434,10.5257560628042,-5.37633860253939));
#30498=CARTESIAN_POINT('Ctrl Pts',(19.5885629966609,10.4626584233998,-5.45734371365233));
#30499=CARTESIAN_POINT('Ctrl Pts',(19.4328211684122,10.3962938213192,-5.5423457101382));
#30500=CARTESIAN_POINT('Ctrl Pts',(19.3101579098382,10.3440246368829,-5.60929382543577));
#30501=CARTESIAN_POINT('Ctrl Pts',(19.1897728266506,10.2897369292767,-5.67868690341334));
#30502=CARTESIAN_POINT('Ctrl Pts',(19.0714153292625,10.2334524706779,-5.75003405792709));
#30503=CARTESIAN_POINT('Ctrl Pts',(18.9016894757456,10.1527399853161,-5.85234660223623));
#30504=CARTESIAN_POINT('Ctrl Pts',(18.7360444326255,10.0678922918024,-5.95870710056834));
#30505=CARTESIAN_POINT('Ctrl Pts',(18.5737726476335,9.9789494966074,-6.06773813254394));
#30506=CARTESIAN_POINT('Ctrl Pts',(18.5595594347906,9.9711590918922,-6.07728804452661));
#30507=CARTESIAN_POINT('Ctrl Pts',(18.5453721176096,9.96333726613753,-6.08685847237853));
#30508=CARTESIAN_POINT('Ctrl Pts',(18.5312102300213,9.95548404389193,-6.09644850639014));
#30509=CARTESIAN_POINT('Ctrl Pts',(18.3626959381603,9.86203744806967,-6.21056166964706));
#30510=CARTESIAN_POINT('Ctrl Pts',(18.1977580193019,9.76404251905382,-6.32756306619599));
#30511=CARTESIAN_POINT('Ctrl Pts',(18.0368078275233,9.66208005126259,-6.44582473286028));
#30512=CARTESIAN_POINT('Ctrl Pts',(17.9197006049216,9.58789224644732,-6.53187182090825));
#30513=CARTESIAN_POINT('Ctrl Pts',(17.8047043242091,9.51160350435421,-6.61858721812569));
#30514=CARTESIAN_POINT('Ctrl Pts',(17.6919753333826,9.43343009819351,-6.70535921700973));
#30515=CARTESIAN_POINT('Ctrl Pts',(17.5883305698321,9.36155626930474,-6.78513872396007));
#30516=CARTESIAN_POINT('Ctrl Pts',(17.4864140067132,9.2879885748002,-6.86510597982913));
#30517=CARTESIAN_POINT('Ctrl Pts',(17.3861179794197,9.21269994086293,-6.94510382222357));
#30518=CARTESIAN_POINT('Ctrl Pts',(17.2254565845855,9.09209718849146,-7.07325012362394));
#30519=CARTESIAN_POINT('Ctrl Pts',(17.0689261099161,8.9670795142694,-7.20146744901835));
#30520=CARTESIAN_POINT('Ctrl Pts',(16.9161092582584,8.83754773326068,-7.32910760378148));
#30521=CARTESIAN_POINT('Ctrl Pts',(16.6930329813764,8.64846212436436,-7.51543188802323));
#30522=CARTESIAN_POINT('Ctrl Pts',(16.4778927674604,8.44975933189865,-7.70056120823172));
#30523=CARTESIAN_POINT('Ctrl Pts',(16.2700797258884,8.24082475266365,-7.88311972782491));
#30524=CARTESIAN_POINT('Ctrl Pts',(16.2451498490466,8.21576033279412,-7.90501999633286));
#30525=CARTESIAN_POINT('Ctrl Pts',(16.2203254556708,8.19054866644283,-7.92688331677123));
#30526=CARTESIAN_POINT('Ctrl Pts',(16.1956055245316,8.16518869245223,-7.94870735251825));
#30527=CARTESIAN_POINT('Ctrl Pts',(16.1143868569095,8.08186712950576,-8.02041139956956));
#30528=CARTESIAN_POINT('Ctrl Pts',(16.0342970299172,7.99694590666152,-8.09169455136918));
#30529=CARTESIAN_POINT('Ctrl Pts',(15.9553273945879,7.91036482251391,-8.16248802407884));
#30530=CARTESIAN_POINT('Ctrl Pts',(15.8085457471954,7.74943569942454,-8.29407255661014));
#30531=CARTESIAN_POINT('Ctrl Pts',(15.6656492987518,7.58280910265095,-8.42393082265112));
#30532=CARTESIAN_POINT('Ctrl Pts',(15.526601377284,7.41012613622904,-8.55162007876201));
#30533=CARTESIAN_POINT('Ctrl Pts',(15.456949520793,7.32362581987266,-8.61558215491674));
#30534=CARTESIAN_POINT('Ctrl Pts',(15.3881779253208,7.23545626402979,-8.67908460554051));
#30535=CARTESIAN_POINT('Ctrl Pts',(15.3204539043479,7.14580024918789,-8.74192602992363));
#30536=CARTESIAN_POINT('Ctrl Pts',(15.2020808298621,6.98909280668051,-8.85176493940411));
#30537=CARTESIAN_POINT('Ctrl Pts',(15.0867965419355,6.82769861550008,-8.95968226768334));
#30538=CARTESIAN_POINT('Ctrl Pts',(14.9755957300485,6.66270594177808,-9.06451837904925));
#30539=CARTESIAN_POINT('Ctrl Pts',(14.9539590767423,6.63060285530961,-9.08491663475525));
#30540=CARTESIAN_POINT('Ctrl Pts',(14.9324769028097,6.59836358094115,-9.10519833700311));
#30541=CARTESIAN_POINT('Ctrl Pts',(14.9111563563958,6.56599618907879,-9.12535509869311));
#30542=CARTESIAN_POINT('Ctrl Pts',(14.8542099711004,6.47954409107802,-9.17919305834126));
#30543=CARTESIAN_POINT('Ctrl Pts',(14.7983371386927,6.39212622784975,-9.23220633207766));
#30544=CARTESIAN_POINT('Ctrl Pts',(14.7435645673992,6.30373776682969,-9.28434781086118));
#30545=CARTESIAN_POINT('Ctrl Pts',(14.6043711417208,6.07911634794631,-9.4168548464161));
#30546=CARTESIAN_POINT('Ctrl Pts',(14.4720730873876,5.84799897797753,-9.54385347643406));
#30547=CARTESIAN_POINT('Ctrl Pts',(14.3469550072385,5.61004377135711,-9.66472083458997));
#30548=CARTESIAN_POINT('Ctrl Pts',(14.2258003780593,5.3796264345101,-9.78175939480288));
#30549=CARTESIAN_POINT('Ctrl Pts',(14.1113780347061,5.14279752758011,-9.89304884696983));
#30550=CARTESIAN_POINT('Ctrl Pts',(14.0039217361569,4.8992787262995,-9.99805135858468));
#30551=CARTESIAN_POINT('Ctrl Pts',(13.966473477019,4.81441301532281,-10.0346444789338));
#30552=CARTESIAN_POINT('Ctrl Pts',(13.9298710234828,4.72873511154457,-10.0704743084635));
#30553=CARTESIAN_POINT('Ctrl Pts',(13.8941235352153,4.64223422283333,-10.105518955736));
#30554=CARTESIAN_POINT('Ctrl Pts',(13.8633808025043,4.56784371793926,-10.135657247299));
#30555=CARTESIAN_POINT('Ctrl Pts',(13.8332549565531,4.49273580938441,-10.1652337840266));
#30556=CARTESIAN_POINT('Ctrl Pts',(13.8037941933816,4.41701904105506,-10.1941954693875));
#30557=CARTESIAN_POINT('Ctrl Pts',(13.7296166127968,4.22637609498908,-10.2671164503283));
#30558=CARTESIAN_POINT('Ctrl Pts',(13.6595331492794,4.03154156271738,-10.3362641811527));
#30559=CARTESIAN_POINT('Ctrl Pts',(13.594367561952,3.83431176397562,-10.4007299350271));
#30560=CARTESIAN_POINT('Ctrl Pts',(13.5639648018699,3.74229494193609,-10.4308061904395));
#30561=CARTESIAN_POINT('Ctrl Pts',(13.5346320185754,3.64975685375333,-10.4598638090668));
#30562=CARTESIAN_POINT('Ctrl Pts',(13.50645002116,3.55687970080345,-10.4878133509968));
#30563=CARTESIAN_POINT('Ctrl Pts',(13.4877362194611,3.49520612255947,-10.5063727943728));
#30564=CARTESIAN_POINT('Ctrl Pts',(13.4695047273751,3.4333370053469,-10.5244681666954));
#30565=CARTESIAN_POINT('Ctrl Pts',(13.4517586041853,3.3712758922898,-10.5420943430048));
#30566=CARTESIAN_POINT('Ctrl Pts',(13.3622742346147,3.05833432655265,-10.6309738835175));
#30567=CARTESIAN_POINT('Ctrl Pts',(13.285027440584,2.74021475838435,-10.7080055004884));
#30568=CARTESIAN_POINT('Ctrl Pts',(13.2203229329071,2.41674037456619,-10.7726649043609));
#30569=CARTESIAN_POINT('Ctrl Pts',(13.2114517859957,2.37239124211817,-10.78152986743));
#30570=CARTESIAN_POINT('Ctrl Pts',(13.2028162317113,2.32794154603814,-10.790162469246));
#30571=CARTESIAN_POINT('Ctrl Pts',(13.1944181700145,2.28339038153381,-10.7985604911309));
#30572=CARTESIAN_POINT('Ctrl Pts',(13.1588819633499,2.09487314432792,-10.8340965293319));
#30573=CARTESIAN_POINT('Ctrl Pts',(13.1276141068245,1.90466457826725,-10.8654110680939));
#30574=CARTESIAN_POINT('Ctrl Pts',(13.1007158995053,1.71250392639037,-10.8923720428026));
#30575=CARTESIAN_POINT('Ctrl Pts',(13.078181338771,1.55151714280708,-10.9149591882885));
#30576=CARTESIAN_POINT('Ctrl Pts',(13.0587141602199,1.38916002469534,-10.9344902732969));
#30577=CARTESIAN_POINT('Ctrl Pts',(13.0423929369339,1.2252700508822,-10.950868868793));
#30578=CARTESIAN_POINT('Ctrl Pts',(13.0400111714759,1.20135349317773,-10.9532590066104));
#30579=CARTESIAN_POINT('Ctrl Pts',(13.0376990687219,1.17741998485909,-10.9555793246671));
#30580=CARTESIAN_POINT('Ctrl Pts',(13.0354566331901,1.15347096186712,-10.9578297968203));
#30581=CARTESIAN_POINT('Ctrl Pts',(13.0191094472756,0.978884390356729,-10.974235569099));
#30582=CARTESIAN_POINT('Ctrl Pts',(13.0064991064528,0.803827357803935,-10.9868998425679));
#30583=CARTESIAN_POINT('Ctrl Pts',(12.9975961675176,0.628791258833778,-10.9958441879377));
#30584=CARTESIAN_POINT('Ctrl Pts',(12.988664151061,0.453183481684936,-11.0048177460648));
#30585=CARTESIAN_POINT('Ctrl Pts',(12.9834637624987,0.27759563306974,-11.0100470817015));
#30586=CARTESIAN_POINT('Ctrl Pts',(12.9820016174814,0.102519509885962,-11.0115175695696));
#30587=CARTESIAN_POINT('Ctrl Pts',(12.98172134674,0.0689601062285234,-11.0117994395073));
#30588=CARTESIAN_POINT('Ctrl Pts',(12.9815785380294,0.0354195213508229,
-11.011943089827));
#30589=CARTESIAN_POINT('Ctrl Pts',(12.9815733914891,0.00190125514371761,
-11.0119482630768));
#30590=CARTESIAN_POINT('Ctrl Pts',(12.9815732941799,0.00126750194249285,
-11.011948360891));
#30591=CARTESIAN_POINT('Ctrl Pts',(12.9815732453836,0.000633750239677955,
-11.0119484099057));
#30592=CARTESIAN_POINT('Ctrl Pts',(12.9815732451008,2.5445788709682E-11,
-11.0119484101204));
#30593=CARTESIAN_POINT('Origin',(23.3621596556826,0.,0.));
#30594=CARTESIAN_POINT('',(32.3980051060631,6.53333333333333,-5.0726277758567));
#30595=CARTESIAN_POINT('Origin',(23.3621596556826,6.53333333333333,0.));
#30596=CARTESIAN_POINT('Ctrl Pts',(32.3980051060631,6.53333333333333,-5.0726277758567));
#30597=CARTESIAN_POINT('Ctrl Pts',(31.8794776108994,7.25152719230469,-5.07127432142549));
#30598=CARTESIAN_POINT('Ctrl Pts',(31.2870113030289,7.89449624331078,-5.06972733998685));
#30599=CARTESIAN_POINT('Ctrl Pts',(30.2913441883522,8.75012170898564,-5.06712608463878));
#30600=CARTESIAN_POINT('Ctrl Pts',(29.9397905959016,9.01808940429159,-5.06620740040415));
#30601=CARTESIAN_POINT('Ctrl Pts',(29.2064698119968,9.51076354319072,-5.06429050665035));
#30602=CARTESIAN_POINT('Ctrl Pts',(28.8285643445812,9.73317788561662,-5.06330239329255));
#30603=CARTESIAN_POINT('Ctrl Pts',(28.0509957610249,10.1317194379082,-5.0612686463517));
#30604=CARTESIAN_POINT('Ctrl Pts',(27.6513307809873,10.3078426825288,-5.06022300812922));
#30605=CARTESIAN_POINT('Ctrl Pts',(26.830050466374,10.6133920770874,-5.05807360020096));
#30606=CARTESIAN_POINT('Ctrl Pts',(26.4058705401804,10.7433739392376,-5.05696311341597));
#30607=CARTESIAN_POINT('Ctrl Pts',(25.1195669733215,11.0550325352827,-5.05359447050841));
#30608=CARTESIAN_POINT('Ctrl Pts',(24.247974768937,11.1600524072644,-5.05131040103342));
#30609=CARTESIAN_POINT('Ctrl Pts',(23.3621596985497,11.1611032573945,-5.04898743093873));
#30610=CARTESIAN_POINT('',(32.3980051060631,-6.53333333333333,-5.07262777585671));
#30611=CARTESIAN_POINT('Ctrl Pts',(23.3622216892987,-11.1611031836844,-5.04898759350387));
#30612=CARTESIAN_POINT('Ctrl Pts',(24.2480154606686,-11.1600475041801,-5.051310507669));
#30613=CARTESIAN_POINT('Ctrl Pts',(25.1195869910657,-11.0550276851818,-5.05359452293198));
#30614=CARTESIAN_POINT('Ctrl Pts',(26.4058705401804,-10.7433739392376,-5.05696311341597));
#30615=CARTESIAN_POINT('Ctrl Pts',(26.830050466374,-10.6133920770874,-5.05807360020097));
#30616=CARTESIAN_POINT('Ctrl Pts',(27.6513307809873,-10.3078426825288,-5.06022300812922));
#30617=CARTESIAN_POINT('Ctrl Pts',(28.0509957610249,-10.1317194379082,-5.0612686463517));
#30618=CARTESIAN_POINT('Ctrl Pts',(28.8285643445811,-9.73317788561662,-5.06330239329256));
#30619=CARTESIAN_POINT('Ctrl Pts',(29.2064698119968,-9.51076354319072,-5.06429050665035));
#30620=CARTESIAN_POINT('Ctrl Pts',(29.9397905959016,-9.01808940429159,-5.06620740040415));
#30621=CARTESIAN_POINT('Ctrl Pts',(30.2913441883522,-8.75012170898565,-5.06712608463878));
#30622=CARTESIAN_POINT('Ctrl Pts',(31.2870113030289,-7.89449624331078,-5.06972733998685));
#30623=CARTESIAN_POINT('Ctrl Pts',(31.8794776108994,-7.2515271923047,-5.07127432142564));
#30624=CARTESIAN_POINT('Ctrl Pts',(32.3980051060631,-6.53333333333333,-5.07262777585671));
#30625=CARTESIAN_POINT('Origin',(23.3621596556826,-6.53333333333334,0.));
#30626=CARTESIAN_POINT('Origin',(-60.4312629272455,0.,0.));
#30627=CARTESIAN_POINT('',(16.3099360798356,-6.,0.));
#30628=CARTESIAN_POINT('',(-60.4312629272455,-6.,0.));
#30629=CARTESIAN_POINT('',(14.1,4.89395944902277E-17,-6.));
#30630=CARTESIAN_POINT('Ctrl Pts',(16.3099360798356,-6.,6.93889390390723E-17));
#30631=CARTESIAN_POINT('Ctrl Pts',(16.3099360798356,-6.,-0.786255652352734));
#30632=CARTESIAN_POINT('Ctrl Pts',(16.1646223990385,-5.83790831484214,-1.59718008826893));
#30633=CARTESIAN_POINT('Ctrl Pts',(15.7042167515933,-5.22042193256505,-3.06257657270413));
#30634=CARTESIAN_POINT('Ctrl Pts',(15.3999322551341,-4.76490888973131,-3.72037248450726));
#30635=CARTESIAN_POINT('Ctrl Pts',(14.8633582506416,-3.72535685789928,-4.75992451633929));
#30636=CARTESIAN_POINT('Ctrl Pts',(14.5899394843239,-3.06638866080029,-5.21878459930749));
#30637=CARTESIAN_POINT('Ctrl Pts',(14.2066217507266,-1.59374871804443,-5.83938521356375));
#30638=CARTESIAN_POINT('Ctrl Pts',(14.1,-0.778751860750423,-6.));
#30639=CARTESIAN_POINT('Ctrl Pts',(14.1,6.93889390390723E-16,-6.));
#30640=CARTESIAN_POINT('',(-3.88784034431744,-7.34788079488412E-16,-6.));
#30641=CARTESIAN_POINT('',(-60.4312629272455,-7.34788079488412E-16,-6.));
#30642=CARTESIAN_POINT('Origin',(-3.88784034431744,0.,0.));
#30643=CARTESIAN_POINT('',(16.3099360798356,6.,0.));
#30644=CARTESIAN_POINT('Ctrl Pts',(14.1,6.93889390390723E-16,-6.));
#30645=CARTESIAN_POINT('Ctrl Pts',(14.1,0.778751860750424,-6.));
#30646=CARTESIAN_POINT('Ctrl Pts',(14.2066217507266,1.59374871804443,-5.83938521356375));
#30647=CARTESIAN_POINT('Ctrl Pts',(14.5899394843239,3.06638866080029,-5.21878459930749));
#30648=CARTESIAN_POINT('Ctrl Pts',(14.8633582506416,3.72535685789928,-4.75992451633929));
#30649=CARTESIAN_POINT('Ctrl Pts',(15.3999322551341,4.76490888973131,-3.72037248450726));
#30650=CARTESIAN_POINT('Ctrl Pts',(15.7042167515933,5.22042193256505,-3.06257657270413));
#30651=CARTESIAN_POINT('Ctrl Pts',(16.1646223990385,5.83790831484214,-1.59718008826893));
#30652=CARTESIAN_POINT('Ctrl Pts',(16.3099360798356,6.,-0.786255652352734));
#30653=CARTESIAN_POINT('Ctrl Pts',(16.3099360798356,6.,0.));
#30654=CARTESIAN_POINT('',(-60.4312629272455,6.,0.));
#30655=CARTESIAN_POINT('Origin',(-3.88784034431744,9.,0.));
#30656=CARTESIAN_POINT('Origin',(31.6603850692973,-6.,0.));
#30657=CARTESIAN_POINT('Origin',(23.35,0.,0.));
#30658=CARTESIAN_POINT('Origin',(31.6603850692973,-6.,0.));
#30659=CARTESIAN_POINT('Origin',(23.35,0.,0.));
#30660=CARTESIAN_POINT('Origin',(23.35,0.,-12.25));
#30661=CARTESIAN_POINT('',(29.8644600669621,-6.56691023510729,-0.418815697553272));
#30662=CARTESIAN_POINT('Ctrl Pts',(23.3560798277625,-9.24999837277875,-1.61173889512423E-9));
#30663=CARTESIAN_POINT('Ctrl Pts',(23.3557691145709,-9.24999837121855,-0.00598343755341071));
#30664=CARTESIAN_POINT('Ctrl Pts',(23.3585014101503,-9.24999612954719,-0.0105107270823176));
#30665=CARTESIAN_POINT('Ctrl Pts',(23.3624176778877,-9.24999071299229,-0.0142079838995739));
#30666=CARTESIAN_POINT('Ctrl Pts',(23.3653670356748,-9.2499866337619,-0.0169924036369621));
#30667=CARTESIAN_POINT('Ctrl Pts',(23.3689921278142,-9.24998075272328,-0.0193042883238705));
#30668=CARTESIAN_POINT('Ctrl Pts',(23.3724772454019,-9.24997260146442,-0.0214104444082658));
#30669=CARTESIAN_POINT('Ctrl Pts',(23.3726619716849,-9.24997216941249,-0.0215220797763884));
#30670=CARTESIAN_POINT('Ctrl Pts',(23.3728462918676,-9.24997173096435,-0.0216331397566146));
#30671=CARTESIAN_POINT('Ctrl Pts',(23.3730300796674,-9.24997128604387,-0.0217436651116202));
#30672=CARTESIAN_POINT('Ctrl Pts',(23.3734340225806,-9.24997030816355,-0.0219865862083058));
#30673=CARTESIAN_POINT('Ctrl Pts',(23.3738353945868,-9.24996929901756,-0.0222269243807324));
#30674=CARTESIAN_POINT('Ctrl Pts',(23.3742328222902,-9.24996825784747,-0.0224651013272281));
#30675=CARTESIAN_POINT('Ctrl Pts',(23.3801893417519,-9.24995265312272,-0.0260348213165618));
#30676=CARTESIAN_POINT('Ctrl Pts',(23.3865182047679,-9.24993006766998,-0.0290684294421575));
#30677=CARTESIAN_POINT('Ctrl Pts',(23.3930123216858,-9.24989993362502,-0.0318040938194547));
#30678=CARTESIAN_POINT('Ctrl Pts',(23.3949401747841,-9.24989098798812,-0.0326162071694723));
#30679=CARTESIAN_POINT('Ctrl Pts',(23.3968823886159,-9.2498813781345,-0.0334023642156201));
#30680=CARTESIAN_POINT('Ctrl Pts',(23.3988330813282,-9.24987109186398,-0.0341694944181134));
#30681=CARTESIAN_POINT('Ctrl Pts',(23.3994515849643,-9.24986783040939,-0.0344127274073939));
#30682=CARTESIAN_POINT('Ctrl Pts',(23.4000705048499,-9.24986450325595,-0.0346538603830449));
#30683=CARTESIAN_POINT('Ctrl Pts',(23.400689667918,-9.24986111021179,-0.0348931350363281));
#30684=CARTESIAN_POINT('Ctrl Pts',(23.4180099648753,-9.24976619412998,-0.0415865382167911));
#30685=CARTESIAN_POINT('Ctrl Pts',(23.4356558940743,-9.24962047407717,-0.0467247754339533));
#30686=CARTESIAN_POINT('Ctrl Pts',(23.4534448814473,-9.24942155576377,-0.0513789487715506));
#30687=CARTESIAN_POINT('Ctrl Pts',(23.454205883255,-9.24941304616214,-0.0515780514100856));
#30688=CARTESIAN_POINT('Ctrl Pts',(23.4549670822585,-9.24940443982341,-0.0517762560936749));
#30689=CARTESIAN_POINT('Ctrl Pts',(23.4557284619145,-9.24939573660621,-0.0519736470538049));
#30690=CARTESIAN_POINT('Ctrl Pts',(23.4918351889383,-9.24898300599922,-0.0613344717854022));
#30691=CARTESIAN_POINT('Ctrl Pts',(23.5284025808039,-9.24835241857728,-0.0685880793220111));
#30692=CARTESIAN_POINT('Ctrl Pts',(23.5651479404171,-9.24749757107013,-0.0751658425167519));
#30693=CARTESIAN_POINT('Ctrl Pts',(23.5660485062986,-9.24747662022064,-0.0753270522360871));
#30694=CARTESIAN_POINT('Ctrl Pts',(23.5669491575448,-9.2474555351634,-0.0754878537145558));
#30695=CARTESIAN_POINT('Ctrl Pts',(23.5678498899729,-9.24743431582261,-0.0756482682765296));
#30696=CARTESIAN_POINT('Ctrl Pts',(23.6420034473011,-9.24568741568394,-0.0888545324753748));
#30697=CARTESIAN_POINT('Ctrl Pts',(23.7165177601391,-9.24303700572992,-0.0990718482177321));
#30698=CARTESIAN_POINT('Ctrl Pts',(23.7910628709197,-9.23947853064399,-0.108338143439424));
#30699=CARTESIAN_POINT('Ctrl Pts',(23.7920741160351,-9.23943025798719,-0.108463845791768));
#30700=CARTESIAN_POINT('Ctrl Pts',(23.7930853619844,-9.23938181845271,-0.108589371555579));
#30701=CARTESIAN_POINT('Ctrl Pts',(23.7940966079193,-9.23933321203489,-0.10871472582196));
#30702=CARTESIAN_POINT('Ctrl Pts',(23.9439866829755,-9.23212861485126,-0.127295132177851));
#30703=CARTESIAN_POINT('Ctrl Pts',(24.094105898176,-9.22125394152026,-0.141687403613213));
#30704=CARTESIAN_POINT('Ctrl Pts',(24.2441262196889,-9.20668443566019,-0.154746477332881));
#30705=CARTESIAN_POINT('Ctrl Pts',(24.2451816356825,-9.2065819369497,-0.154838349921378));
#30706=CARTESIAN_POINT('Ctrl Pts',(24.2462370466876,-9.20647925543194,-0.154930156309389));
#30707=CARTESIAN_POINT('Ctrl Pts',(24.2472924526095,-9.20637639109876,-0.155021897491501));
#30708=CARTESIAN_POINT('Ctrl Pts',(24.5482990564597,-9.17703901204522,-0.181186902906664));
#30709=CARTESIAN_POINT('Ctrl Pts',(24.8468428326049,-9.13300625249746,-0.201286064954757));
#30710=CARTESIAN_POINT('Ctrl Pts',(25.1409132619702,-9.07497270906441,-0.219347970745817));
#30711=CARTESIAN_POINT('Ctrl Pts',(25.1418786391976,-9.07478219599115,-0.219407264543468));
#30712=CARTESIAN_POINT('Ctrl Pts',(25.1428439684873,-9.07459153201271,-0.219466536374313));
#30713=CARTESIAN_POINT('Ctrl Pts',(25.1438092497709,-9.07440071715349,-0.219525786380926));
#30714=CARTESIAN_POINT('Ctrl Pts',(25.6986244953389,-8.96472595730263,-0.253580944731915));
#30715=CARTESIAN_POINT('Ctrl Pts',(26.2398207194525,-8.80535458783623,-0.2798503572218));
#30716=CARTESIAN_POINT('Ctrl Pts',(26.7669586035649,-8.59575408308744,-0.303211664728421));
#30717=CARTESIAN_POINT('Ctrl Pts',(26.7996081847069,-8.58277196039532,-0.304658604756847));
#30718=CARTESIAN_POINT('Ctrl Pts',(26.8322038387004,-8.56959716131495,-0.306094393823134));
#30719=CARTESIAN_POINT('Ctrl Pts',(26.8647454628159,-8.55622956530362,-0.307520192718601));
#30720=CARTESIAN_POINT('Ctrl Pts',(26.8654093710352,-8.55595684207283,-0.307549281604956));
#30721=CARTESIAN_POINT('Ctrl Pts',(26.8660732568065,-8.55568403857651,-0.307578366327974));
#30722=CARTESIAN_POINT('Ctrl Pts',(26.8667371201291,-8.55541115481362,-0.307607446897494));
#30723=CARTESIAN_POINT('Ctrl Pts',(27.1454796620206,-8.44083288074899,-0.319817779345406));
#30724=CARTESIAN_POINT('Ctrl Pts',(27.4215277388667,-8.31121170489241,-0.331185606618138));
#30725=CARTESIAN_POINT('Ctrl Pts',(27.6880931473778,-8.16966632158923,-0.341697123203151));
#30726=CARTESIAN_POINT('Ctrl Pts',(27.6885803173162,-8.16940763590281,-0.341716333853613));
#30727=CARTESIAN_POINT('Ctrl Pts',(27.6890674556256,-8.16914891036779,-0.341735541645787));
#30728=CARTESIAN_POINT('Ctrl Pts',(27.6895545622644,-8.16889014500319,-0.341754746579587));
#30729=CARTESIAN_POINT('Ctrl Pts',(27.9562330077065,-8.02722271600935,-0.352268957396166));
#30730=CARTESIAN_POINT('Ctrl Pts',(28.2143884397778,-7.87337926937015,-0.361969675425041));
#30731=CARTESIAN_POINT('Ctrl Pts',(28.4641910486503,-7.70762933209229,-0.371041147542007));
#30732=CARTESIAN_POINT('Ctrl Pts',(28.4645007674479,-7.7074238263472,-0.371052394844221));
#30733=CARTESIAN_POINT('Ctrl Pts',(28.4648104733983,-7.70721830230421,-0.371063641178871));
#30734=CARTESIAN_POINT('Ctrl Pts',(28.4651201665019,-7.70701275996383,-0.371074886546309));
#30735=CARTESIAN_POINT('Ctrl Pts',(28.9095707576435,-7.41203229832873,-0.387213477126958));
#30736=CARTESIAN_POINT('Ctrl Pts',(29.327778597325,-7.07962587936707,-0.401386883213377));
#30737=CARTESIAN_POINT('Ctrl Pts',(29.7187223777706,-6.70836707619969,-0.414101709608085));
#30738=CARTESIAN_POINT('Ctrl Pts',(29.767730781015,-6.66182636614427,-0.415695630192842));
#30739=CARTESIAN_POINT('Ctrl Pts',(29.8163106926773,-6.61467503846194,-0.417266627326651));
#30740=CARTESIAN_POINT('Ctrl Pts',(29.8644600669621,-6.56691023510729,-0.418815697553251));
#30741=CARTESIAN_POINT('',(30.4989465761475,-5.86984351166102,-2.5869876306867));
#30742=CARTESIAN_POINT('Ctrl Pts',(29.8644600669621,-6.56691023510729,-0.418815697553272));
#30743=CARTESIAN_POINT('Ctrl Pts',(29.8733746637293,-6.55806683957206,-0.419102499544775));
#30744=CARTESIAN_POINT('Ctrl Pts',(29.8810061889829,-6.55046075135664,-0.426908455290693));
#30745=CARTESIAN_POINT('Ctrl Pts',(29.8934944746253,-6.53798577209718,-0.444265632584569));
#30746=CARTESIAN_POINT('Ctrl Pts',(29.8987214649284,-6.53274778761039,-0.454306399100273));
#30747=CARTESIAN_POINT('Ctrl Pts',(29.9131557521886,-6.51825686050047,-0.485213053623094));
#30748=CARTESIAN_POINT('Ctrl Pts',(29.9211884729116,-6.51015350884117,-0.507262215490086));
#30749=CARTESIAN_POINT('Ctrl Pts',(29.9439661829232,-6.48710849294812,-0.574043018301807));
#30750=CARTESIAN_POINT('Ctrl Pts',(29.9572126448329,-6.47360662755049,-0.619820775336012));
#30751=CARTESIAN_POINT('Ctrl Pts',(29.9959438791152,-6.43391768402986,-0.757554586253613));
#30752=CARTESIAN_POINT('Ctrl Pts',(30.0200501387962,-6.40891263751482,-0.850295961307722));
#30753=CARTESIAN_POINT('Ctrl Pts',(30.0926610277737,-6.33276736205838,-1.12809260388518));
#30754=CARTESIAN_POINT('Ctrl Pts',(30.1409280530889,-6.28101981664688,-1.31302684036839));
#30755=CARTESIAN_POINT('Ctrl Pts',(30.2895149536044,-6.11778450470958,-1.86433248511176));
#30756=CARTESIAN_POINT('Ctrl Pts',(30.3930163475332,-5.99885709501432,-2.22754310454855));
#30757=CARTESIAN_POINT('Ctrl Pts',(30.4989465761475,-5.86984351166102,-2.5869876306867));
#30758=CARTESIAN_POINT('',(30.8496157942439,-5.41463414634147,-3.60555127546399));
#30759=CARTESIAN_POINT('Ctrl Pts',(30.4989465761475,-5.86984351166102,-2.5869876306867));
#30760=CARTESIAN_POINT('Ctrl Pts',(30.5547782956591,-5.80184545017096,-2.7764369102171));
#30761=CARTESIAN_POINT('Ctrl Pts',(30.6146971569704,-5.72690380650632,-2.96137640232734));
#30762=CARTESIAN_POINT('Ctrl Pts',(30.677808767019,-5.64497703242559,-3.14209440617126));
#30763=CARTESIAN_POINT('Ctrl Pts',(30.7328569315897,-5.57351762045888,-3.29972300111334));
#30764=CARTESIAN_POINT('Ctrl Pts',(30.7903333826036,-5.49674409110279,-3.45414026184368));
#30765=CARTESIAN_POINT('Ctrl Pts',(30.8496157942439,-5.41463414634147,-3.60555127546398));
#30766=CARTESIAN_POINT('',(30.8496157942439,-5.41463414634147,-4.65853571252147));
#30767=CARTESIAN_POINT('',(30.8496157942439,-5.41463414634147,-12.25));
#30768=CARTESIAN_POINT('',(23.4134558714741,-9.24978690988232,-4.63699261464813));
#30769=CARTESIAN_POINT('Ctrl Pts',(30.8496157942439,-5.41463414634147,-4.65853571252147));
#30770=CARTESIAN_POINT('Ctrl Pts',(30.4224818233768,-6.00624210868884,-4.65730028266087));
#30771=CARTESIAN_POINT('Ctrl Pts',(29.9348006057638,-6.5362496484837,-4.65588924421514));
#30772=CARTESIAN_POINT('Ctrl Pts',(29.1157096677008,-7.24216864268045,-4.65351797766776));
#30773=CARTESIAN_POINT('Ctrl Pts',(28.8267164809711,-7.46328115931847,-4.65268114057206));
#30774=CARTESIAN_POINT('Ctrl Pts',(28.2233249304723,-7.87055863316035,-4.65093338408782));
#30775=CARTESIAN_POINT('Ctrl Pts',(27.9124127490458,-8.05459039487177,-4.65003256384235));
#30776=CARTESIAN_POINT('Ctrl Pts',(27.2727683495141,-8.38474358569576,-4.64817872235552));
#30777=CARTESIAN_POINT('Ctrl Pts',(26.9440345067492,-8.53086155850978,-4.6472256966148));
#30778=CARTESIAN_POINT('Ctrl Pts',(26.2686099494916,-8.78489606818956,-4.64526695104862));
#30779=CARTESIAN_POINT('Ctrl Pts',(25.9199435996119,-8.89326151785136,-4.64425549764083));
#30780=CARTESIAN_POINT('Ctrl Pts',(24.8609128854777,-9.15469739384237,-4.64118229168174));
#30781=CARTESIAN_POINT('Ctrl Pts',(24.1431288109746,-9.24477620324171,-4.63909799546489));
#30782=CARTESIAN_POINT('Ctrl Pts',(23.4134608743401,-9.24978230648852,-4.63697771328011));
#30783=CARTESIAN_POINT('',(23.4134609280924,9.249790502254,-4.63697771320315));
#30784=CARTESIAN_POINT('Ctrl Pts',(23.4134536511895,-9.24977205774196,-4.63699888793905));
#30785=CARTESIAN_POINT('Ctrl Pts',(23.3625154232152,-9.25012518184601,-4.6198065222011));
#30786=CARTESIAN_POINT('Ctrl Pts',(23.3113786668813,-9.25006107462989,-4.6034901913981));
#30787=CARTESIAN_POINT('Ctrl Pts',(23.2601805794695,-9.24956390714826,-4.58816205258291));
#30788=CARTESIAN_POINT('Ctrl Pts',(23.0981361101497,-9.24799034757217,-4.53964773797597));
#30789=CARTESIAN_POINT('Ctrl Pts',(22.9348134041621,-9.24215350764586,-4.50067157209841));
#30790=CARTESIAN_POINT('Ctrl Pts',(22.7699677329688,-9.23179628076355,-4.47253333001147));
#30791=CARTESIAN_POINT('Ctrl Pts',(22.6606958452985,-9.22493074571938,-4.45388122464344));
#30792=CARTESIAN_POINT('Ctrl Pts',(22.5507538239542,-9.21607845109921,-4.43999863426792));
#30793=CARTESIAN_POINT('Ctrl Pts',(22.4400833769471,-9.20513819700547,-4.43119193287283));
#30794=CARTESIAN_POINT('Ctrl Pts',(22.3843570454958,-9.19962940724021,-4.42675745940491));
#30795=CARTESIAN_POINT('Ctrl Pts',(22.3283580105308,-9.1935818903447,-4.42360382581514));
#30796=CARTESIAN_POINT('Ctrl Pts',(22.2721719172255,-9.18699007422903,-4.42178202558678));
#30797=CARTESIAN_POINT('Ctrl Pts',(22.1990930360943,-9.17841637710902,-4.41941248688955));
#30798=CARTESIAN_POINT('Ctrl Pts',(22.1257309771798,-9.16890595979547,-4.41934771320976));
#30799=CARTESIAN_POINT('Ctrl Pts',(22.0527227559231,-9.15856206490708,-4.42150072981427));
#30800=CARTESIAN_POINT('Ctrl Pts',(22.0154729646368,-9.153284468507,-4.42259922828161));
#30801=CARTESIAN_POINT('Ctrl Pts',(21.9783152749303,-9.14779021638894,-4.42427425890002));
#30802=CARTESIAN_POINT('Ctrl Pts',(21.9413331248964,-9.14209478477932,-4.42650949742667));
#30803=CARTESIAN_POINT('Ctrl Pts',(21.8845228329765,-9.13334572254104,-4.42994316888961));
#30804=CARTESIAN_POINT('Ctrl Pts',(21.8279757871699,-9.12409883599493,-4.43470752363319));
#30805=CARTESIAN_POINT('Ctrl Pts',(21.7719128739377,-9.11439197218095,-4.4407627349337));
#30806=CARTESIAN_POINT('Ctrl Pts',(21.6649547696481,-9.09587299604709,-4.45231500513226));
#30807=CARTESIAN_POINT('Ctrl Pts',(21.5591625981775,-9.0756190286987,-4.46851612585592));
#30808=CARTESIAN_POINT('Ctrl Pts',(21.454548075228,-9.0537166137703,-4.48890446567054));
#30809=CARTESIAN_POINT('Ctrl Pts',(21.3980429074417,-9.041886519864,-4.49991676615835));
#30810=CARTESIAN_POINT('Ctrl Pts',(21.3418595080924,-9.02957122376613,-4.51215442073769));
#30811=CARTESIAN_POINT('Ctrl Pts',(21.2859920296565,-9.01678274654428,-4.52554647006272));
#30812=CARTESIAN_POINT('Ctrl Pts',(21.1261165989934,-8.98018608314352,-4.56387036999955));
#30813=CARTESIAN_POINT('Ctrl Pts',(20.968827586669,-8.93971141831164,-4.61163882662143));
#30814=CARTESIAN_POINT('Ctrl Pts',(20.8139926873238,-8.89557007225076,-4.66712904960507));
#30815=CARTESIAN_POINT('Ctrl Pts',(20.7175752575018,-8.8680827605783,-4.70168343432688));
#30816=CARTESIAN_POINT('Ctrl Pts',(20.6227601556529,-8.83935856288174,-4.73899129256353));
#30817=CARTESIAN_POINT('Ctrl Pts',(20.5295418854412,-8.80951347275127,-4.77853066159051));
#30818=CARTESIAN_POINT('Ctrl Pts',(20.4722797482889,-8.79118022498244,-4.80281891288497));
#30819=CARTESIAN_POINT('Ctrl Pts',(20.415594740856,-8.77241599294277,-4.82796055678945));
#30820=CARTESIAN_POINT('Ctrl Pts',(20.3594786464077,-8.75324408626673,-4.85384151791365));
#30821=CARTESIAN_POINT('Ctrl Pts',(20.2112845228144,-8.70261397853378,-4.9221892243829));
#30822=CARTESIAN_POINT('Ctrl Pts',(20.0668379773865,-8.64907446285856,-4.99577768538368));
#30823=CARTESIAN_POINT('Ctrl Pts',(19.9255222376653,-8.59275578941024,-5.07319877354532));
#30824=CARTESIAN_POINT('Ctrl Pts',(19.8444601752456,-8.56045006160199,-5.11760934729691));
#30825=CARTESIAN_POINT('Ctrl Pts',(19.7643251743023,-8.52718104617017,-5.16333201725847));
#30826=CARTESIAN_POINT('Ctrl Pts',(19.6851507542395,-8.49301403080143,-5.21011167025964));
#30827=CARTESIAN_POINT('Ctrl Pts',(19.5204367414571,-8.42193316653096,-5.30743179406061));
#30828=CARTESIAN_POINT('Ctrl Pts',(19.3594003020667,-8.34675420139556,-5.40956187554908));
#30829=CARTESIAN_POINT('Ctrl Pts',(19.2025571830132,-8.26808276251442,-5.51423100984347));
#30830=CARTESIAN_POINT('Ctrl Pts',(19.1705496927634,-8.25202802368925,-5.53559118372682));
#30831=CARTESIAN_POINT('Ctrl Pts',(19.1387167227146,-8.2358279579899,-5.55705704428414));
#30832=CARTESIAN_POINT('Ctrl Pts',(19.1070624667525,-8.21948788514045,-5.57860925559438));
#30833=CARTESIAN_POINT('Ctrl Pts',(19.040072240914,-8.1849072217468,-5.62422042095298));
#30834=CARTESIAN_POINT('Ctrl Pts',(18.973874871607,-8.14970640323712,-5.67021831303887));
#30835=CARTESIAN_POINT('Ctrl Pts',(18.9084396350559,-8.11389278588748,-5.71652425076615));
#30836=CARTESIAN_POINT('Ctrl Pts',(18.7176376007028,-8.00946417207001,-5.85154732986952));
#30837=CARTESIAN_POINT('Ctrl Pts',(18.5329968378859,-7.89965487887584,-5.98927781427906));
#30838=CARTESIAN_POINT('Ctrl Pts',(18.3533564211586,-7.78434666162082,-6.12812846959049));
#30839=CARTESIAN_POINT('Ctrl Pts',(18.2996301970183,-7.74986068547852,-6.16965543532115));
#30840=CARTESIAN_POINT('Ctrl Pts',(18.2463541938633,-7.71488252716231,-6.2112866342043));
#30841=CARTESIAN_POINT('Ctrl Pts',(18.1935123904376,-7.67940451382411,-6.25299729234993));
#30842=CARTESIAN_POINT('Ctrl Pts',(18.0087538346775,-7.55535752676715,-6.39883639054874));
#30843=CARTESIAN_POINT('Ctrl Pts',(17.8292147797447,-7.42513966469565,-6.54564052692412));
#30844=CARTESIAN_POINT('Ctrl Pts',(17.6543191662457,-7.28846484833837,-6.69218578884888));
#30845=CARTESIAN_POINT('Ctrl Pts',(17.4293790572173,-7.11268200577425,-6.88066339863838));
#30846=CARTESIAN_POINT('Ctrl Pts',(17.2121426350658,-6.92622255174211,-7.0687519212596));
#30847=CARTESIAN_POINT('Ctrl Pts',(17.0021480411652,-6.72809597948268,-7.25458119189773));
#30848=CARTESIAN_POINT('Ctrl Pts',(16.9697452200666,-6.69752443115584,-7.28325522821234));
#30849=CARTESIAN_POINT('Ctrl Pts',(16.9374967681784,-6.66665407851879,-7.3118928664918));
#30850=CARTESIAN_POINT('Ctrl Pts',(16.9054125928198,-6.63549059697695,-7.34047940783783));
#30851=CARTESIAN_POINT('Ctrl Pts',(16.7671279762097,-6.50117422296744,-7.463689023359));
#30852=CARTESIAN_POINT('Ctrl Pts',(16.6316353181641,-6.36115478230237,-7.58616693585297));
#30853=CARTESIAN_POINT('Ctrl Pts',(16.4998949000094,-6.21598638326824,-7.70660105121202));
#30854=CARTESIAN_POINT('Ctrl Pts',(16.4643815647232,-6.17685325996352,-7.73906654038045));
#30855=CARTESIAN_POINT('Ctrl Pts',(16.4291407972998,-6.137346246477,-7.77138348493443));
#30856=CARTESIAN_POINT('Ctrl Pts',(16.3941911402224,-6.09747678193591,-7.80352619206129));
#30857=CARTESIAN_POINT('Ctrl Pts',(16.3704901831911,-6.07043947899866,-7.82532362826506));
#30858=CARTESIAN_POINT('Ctrl Pts',(16.346936709246,-6.04325350110009,-7.84702809310363));
#30859=CARTESIAN_POINT('Ctrl Pts',(16.3235317154403,-6.01591845087238,-7.86863650241515));
#30860=CARTESIAN_POINT('Ctrl Pts',(16.1552502807965,-5.81937998961162,-8.02400053068656));
#30861=CARTESIAN_POINT('Ctrl Pts',(15.9944684313001,-5.6149337711535,-8.17456347625085));
#30862=CARTESIAN_POINT('Ctrl Pts',(15.8412586152749,-5.40197212305963,-8.31941227715205));
#30863=CARTESIAN_POINT('Ctrl Pts',(15.8251737266489,-5.3796141274685,-8.33461937608707));
#30864=CARTESIAN_POINT('Ctrl Pts',(15.8091710738808,-5.35716349022867,-8.34976430237018));
#30865=CARTESIAN_POINT('Ctrl Pts',(15.7932513756019,-5.33461898106988,-8.36484577448847));
#30866=CARTESIAN_POINT('Ctrl Pts',(15.6711357265184,-5.16168622060058,-8.48053162007448));
#30867=CARTESIAN_POINT('Ctrl Pts',(15.5539386693611,-4.98328907382023,-8.59246306301524));
#30868=CARTESIAN_POINT('Ctrl Pts',(15.4419436637423,-4.7988015802883,-8.70010725775847));
#30869=CARTESIAN_POINT('Ctrl Pts',(15.3349318152216,-4.62252275782897,-8.80296188237635));
#30870=CARTESIAN_POINT('Ctrl Pts',(15.2326693884291,-4.44068357906781,-8.90190244898871));
#30871=CARTESIAN_POINT('Ctrl Pts',(15.135429249196,-4.25270849650674,-8.99643824681075));
#30872=CARTESIAN_POINT('Ctrl Pts',(15.0615819586205,-4.10995417044033,-9.06823177350253));
#30873=CARTESIAN_POINT('Ctrl Pts',(14.9906316960674,-3.96366048599508,-9.13748442942233));
#30874=CARTESIAN_POINT('Ctrl Pts',(14.9227086452196,-3.81356269417404,-9.20396968784947));
#30875=CARTESIAN_POINT('Ctrl Pts',(14.9168048317238,-3.80051632246408,-9.20974852965753));
#30876=CARTESIAN_POINT('Ctrl Pts',(14.9109288888533,-3.78745181862973,-9.2155015917612));
#30877=CARTESIAN_POINT('Ctrl Pts',(14.9050809147943,-3.77436910755354,-9.2212287385584));
#30878=CARTESIAN_POINT('Ctrl Pts',(14.8094865402887,-3.56051152721262,-9.31484800058859));
#30879=CARTESIAN_POINT('Ctrl Pts',(14.7215332654277,-3.34217122454843,-9.40138352891765));
#30880=CARTESIAN_POINT('Ctrl Pts',(14.6415966822654,-3.11908192459304,-9.48029264021483));
#30881=CARTESIAN_POINT('Ctrl Pts',(14.5642383968141,-2.90318821154769,-9.55665659417615));
#30882=CARTESIAN_POINT('Ctrl Pts',(14.4943879619239,-2.68284690098548,-9.62587828797752));
#30883=CARTESIAN_POINT('Ctrl Pts',(14.432417365367,-2.45780017141991,-9.68743324706195));
#30884=CARTESIAN_POINT('Ctrl Pts',(14.3893243216042,-2.30130742962521,-9.73023726530642));
#30885=CARTESIAN_POINT('Ctrl Pts',(14.350042231419,-2.14253903782754,-9.76933335602689));
#30886=CARTESIAN_POINT('Ctrl Pts',(14.3147058328292,-1.98140336961855,-9.8045348690398));
#30887=CARTESIAN_POINT('Ctrl Pts',(14.3136044543346,-1.97638103098872,-9.80563204336872));
#30888=CARTESIAN_POINT('Ctrl Pts',(14.31250696286,-1.97135599428855,-9.80672539075607));
#30889=CARTESIAN_POINT('Ctrl Pts',(14.3114133683192,-1.96632830061353,-9.80781490049638));
#30890=CARTESIAN_POINT('Ctrl Pts',(14.2745987957367,-1.79707691281701,-9.844491963079));
#30891=CARTESIAN_POINT('Ctrl Pts',(14.2421976357723,-1.62478683090103,-9.87681844509401));
#30892=CARTESIAN_POINT('Ctrl Pts',(14.2146208502178,-1.45124442493548,-9.90435663415071));
#30893=CARTESIAN_POINT('Ctrl Pts',(14.1905893369956,-1.30001263559869,-9.92835451284191));
#30894=CARTESIAN_POINT('Ctrl Pts',(14.1702212471377,-1.14783143755459,-9.94871632506298));
#30895=CARTESIAN_POINT('Ctrl Pts',(14.1537676058962,-0.995896457287379,
-9.9651728621265));
#30896=CARTESIAN_POINT('Ctrl Pts',(14.1535154766557,-0.993568264358871,
-9.9654250357415));
#30897=CARTESIAN_POINT('Ctrl Pts',(14.1532642330707,-0.991240013867564,
-9.96567632576613));
#30898=CARTESIAN_POINT('Ctrl Pts',(14.1530138752056,-0.988911706202816,
-9.96592673211944));
#30899=CARTESIAN_POINT('Ctrl Pts',(14.1176771446479,-0.660283002753475,
-10.0012703065398));
#30900=CARTESIAN_POINT('Ctrl Pts',(14.0999586550532,-0.330265416703061,
-10.0190270165079));
#30901=CARTESIAN_POINT('Ctrl Pts',(14.1000000720546,0.00115476959212982,
-10.0189855634338));
#30902=CARTESIAN_POINT('Ctrl Pts',(14.1000000889788,0.00129019738339432,
-10.0189855464949));
#30903=CARTESIAN_POINT('Ctrl Pts',(14.1000001088685,0.00142562543411628,
-10.0189855265846));
#30904=CARTESIAN_POINT('Ctrl Pts',(14.1000001317237,0.00156105374426756,
-10.0189855037028));
#30905=CARTESIAN_POINT('Ctrl Pts',(14.1000358072751,0.212955982700576,-10.0189497867261));
#30906=CARTESIAN_POINT('Ctrl Pts',(14.1074048420233,0.425862245288223,-10.0115660274281));
#30907=CARTESIAN_POINT('Ctrl Pts',(14.122083690801,0.638308793476026,-9.99687450483632));
#30908=CARTESIAN_POINT('Ctrl Pts',(14.1304086932907,0.758796310539954,-9.98854231448503));
#30909=CARTESIAN_POINT('Ctrl Pts',(14.1410842316643,0.879135733516061,-9.97786025043846));
#30910=CARTESIAN_POINT('Ctrl Pts',(14.1541007419723,0.998967596774582,-9.96484091674184));
#30911=CARTESIAN_POINT('Ctrl Pts',(14.1543587496805,1.00134285279034,-9.9645828530696));
#30912=CARTESIAN_POINT('Ctrl Pts',(14.1546176737308,1.00371787914823,-9.96432387482324));
#30913=CARTESIAN_POINT('Ctrl Pts',(14.1548775139933,1.00609267334345,-9.96406398215856));
#30914=CARTESIAN_POINT('Ctrl Pts',(14.1811166565157,1.24590371242471,-9.937819547971));
#30915=CARTESIAN_POINT('Ctrl Pts',(14.2163411509945,1.48142568176268,-9.90260913254167));
#30916=CARTESIAN_POINT('Ctrl Pts',(14.2599907469931,1.71300461953484,-9.85906875646823));
#30917=CARTESIAN_POINT('Ctrl Pts',(14.2761915859853,1.79895668848331,-9.84290845518043));
#30918=CARTESIAN_POINT('Ctrl Pts',(14.2935533937762,1.88436542320633,-9.82560027869732));
#30919=CARTESIAN_POINT('Ctrl Pts',(14.3120487231286,1.96924799329246,-9.80717550881918));
#30920=CARTESIAN_POINT('Ctrl Pts',(14.313179333629,1.97443682357576,-9.80604921158513));
#30921=CARTESIAN_POINT('Ctrl Pts',(14.3143141770252,1.97962367355132,-9.80491874382379));
#30922=CARTESIAN_POINT('Ctrl Pts',(14.3154532468789,1.98480854635299,-9.8037841128692));
#30923=CARTESIAN_POINT('Ctrl Pts',(14.3836494945956,2.29522749810616,-9.73585362257075));
#30924=CARTESIAN_POINT('Ctrl Pts',(14.4670033588811,2.59855545823469,-9.6529906171091));
#30925=CARTESIAN_POINT('Ctrl Pts',(14.5647724800604,2.89521670871526,-9.55625712062353));
#30926=CARTESIAN_POINT('Ctrl Pts',(14.5677239339626,2.90417231754967,-9.5533369301561));
#30927=CARTESIAN_POINT('Ctrl Pts',(14.5706885923883,2.91312204824748,-9.55040404547431));
#30928=CARTESIAN_POINT('Ctrl Pts',(14.5736664294657,2.92206588883981,-9.5474584999236));
#30929=CARTESIAN_POINT('Ctrl Pts',(14.6311104426171,3.09459718698157,-9.4906374069767));
#30930=CARTESIAN_POINT('Ctrl Pts',(14.6937223783733,3.26537270008771,-9.42884780434795));
#30931=CARTESIAN_POINT('Ctrl Pts',(14.7605830856977,3.4327015772179,-9.36307478257347));
#30932=CARTESIAN_POINT('Ctrl Pts',(14.8069875664328,3.54883570091995,-9.31742520685158));
#30933=CARTESIAN_POINT('Ctrl Pts',(14.8554380267574,3.66331003509001,-9.26985741257131));
#30934=CARTESIAN_POINT('Ctrl Pts',(14.9056220961044,3.77557290469752,-9.22070457934102));
#30935=CARTESIAN_POINT('Ctrl Pts',(14.9115531749302,3.78884085880157,-9.21489537868846));
#30936=CARTESIAN_POINT('Ctrl Pts',(14.9175089427579,3.80207900624528,-9.20906364098573));
#30937=CARTESIAN_POINT('Ctrl Pts',(14.9234889314797,3.8152865178915,-9.2032098747074));
#30938=CARTESIAN_POINT('Ctrl Pts',(15.0533909246116,4.10219041804352,-9.07604978423608));
#30939=CARTESIAN_POINT('Ctrl Pts',(15.1950267960996,4.37660230577789,-8.9381228709984));
#30940=CARTESIAN_POINT('Ctrl Pts',(15.3475682128899,4.63969858186413,-8.79097067465315));
#30941=CARTESIAN_POINT('Ctrl Pts',(15.4869290652399,4.88006163903903,-8.65653337926571));
#30942=CARTESIAN_POINT('Ctrl Pts',(15.6353925190135,5.11097971039312,-8.5143956859272));
#30943=CARTESIAN_POINT('Ctrl Pts',(15.7923412757554,5.33332861190327,-8.36570498428764));
#30944=CARTESIAN_POINT('Ctrl Pts',(15.8085748204292,5.35632663304574,-8.35032558786711));
#30945=CARTESIAN_POINT('Ctrl Pts',(15.8249007586485,5.37923523180617,-8.33487457054184));
#30946=CARTESIAN_POINT('Ctrl Pts',(15.841318190271,5.40205493130655,-8.3193533874901));
#30947=CARTESIAN_POINT('Ctrl Pts',(15.9564445782044,5.56207689074639,-8.21051189618467));
#30948=CARTESIAN_POINT('Ctrl Pts',(16.0764315943577,5.7179387366289,-8.09791750495548));
#30949=CARTESIAN_POINT('Ctrl Pts',(16.199859969054,5.86835059952874,-7.98321179303217));
#30950=CARTESIAN_POINT('Ctrl Pts',(16.2413376889731,5.91889603640444,-7.94466529670187));
#30951=CARTESIAN_POINT('Ctrl Pts',(16.2832039606803,5.96882642578861,-7.90588033707161));
#30952=CARTESIAN_POINT('Ctrl Pts',(16.3254048483401,6.01809418238744,-7.86691892834382));
#30953=CARTESIAN_POINT('Ctrl Pts',(16.3490689997507,6.04572108116765,-7.84507131502498));
#30954=CARTESIAN_POINT('Ctrl Pts',(16.3728474309111,6.07315021492223,-7.82316039810069));
#30955=CARTESIAN_POINT('Ctrl Pts',(16.3967310211233,6.10037298103729,-7.80119685223178));
#30956=CARTESIAN_POINT('Ctrl Pts',(16.5406119366081,6.26436995451789,-7.66888277973158));
#30957=CARTESIAN_POINT('Ctrl Pts',(16.6887165728628,6.42152235603342,-7.53425782398027));
#30958=CARTESIAN_POINT('Ctrl Pts',(16.8408982921417,6.5722306611734,-7.39807639652365));
#30959=CARTESIAN_POINT('Ctrl Pts',(16.8616786155221,6.59280979072818,-7.3794809034884));
#30960=CARTESIAN_POINT('Ctrl Pts',(16.8825349128291,6.61326882820459,-7.36085640205674));
#30961=CARTESIAN_POINT('Ctrl Pts',(16.9034667668706,6.63360885105693,-7.34220482308772));
#30962=CARTESIAN_POINT('Ctrl Pts',(16.9356171064303,6.66485016585206,-7.3135568783815));
#30963=CARTESIAN_POINT('Ctrl Pts',(16.9679485682156,6.69581350788118,-7.28484298464478));
#30964=CARTESIAN_POINT('Ctrl Pts',(17.0004614301616,6.72650428901826,-7.25606858825597));
#30965=CARTESIAN_POINT('Ctrl Pts',(17.196485101874,6.91154243226739,-7.08258454244043));
#30966=CARTESIAN_POINT('Ctrl Pts',(17.3990929751407,7.08666865088716,-6.90688154140969));
#30967=CARTESIAN_POINT('Ctrl Pts',(17.6088306131168,7.25268813035639,-6.7303865509183));
#30968=CARTESIAN_POINT('Ctrl Pts',(17.6227451945787,7.26370232691938,-6.71867737965797));
#30969=CARTESIAN_POINT('Ctrl Pts',(17.6366911658378,7.27467642584925,-6.70696471709683));
#30970=CARTESIAN_POINT('Ctrl Pts',(17.6506686901954,7.28561065581231,-6.69524897787459));
#30971=CARTESIAN_POINT('Ctrl Pts',(17.8251083620105,7.42206997704129,-6.54903641170733));
#30972=CARTESIAN_POINT('Ctrl Pts',(18.0044456079559,7.55231948063633,-6.40232005328148));
#30973=CARTESIAN_POINT('Ctrl Pts',(18.1893889970805,7.67663444272538,-6.25626363447874));
#30974=CARTESIAN_POINT('Ctrl Pts',(18.2427346090674,7.7124922139231,-6.21413469392824));
#30975=CARTESIAN_POINT('Ctrl Pts',(18.2965462682594,7.74785583569029,-6.1720651548733));
#30976=CARTESIAN_POINT('Ctrl Pts',(18.3508438446585,7.78273330775818,-6.13008043092315));
#30977=CARTESIAN_POINT('Ctrl Pts',(18.5142781265021,7.88771358455781,-6.0037075122362));
#30978=CARTESIAN_POINT('Ctrl Pts',(18.6826314570586,7.98854931917481,-5.87771460460918));
#30979=CARTESIAN_POINT('Ctrl Pts',(18.8553464773727,8.08457873025275,-5.7543318478112));
#30980=CARTESIAN_POINT('Ctrl Pts',(18.9386356116647,8.13088742130181,-5.69483243090129));
#30981=CARTESIAN_POINT('Ctrl Pts',(19.0229393625003,8.176077953008,-5.63594037502953));
#30982=CARTESIAN_POINT('Ctrl Pts',(19.1081966589314,8.22007326509797,-5.57790904883187));
#30983=CARTESIAN_POINT('Ctrl Pts',(19.260373168651,8.2986008905112,-5.47432841650077));
#30984=CARTESIAN_POINT('Ctrl Pts',(19.4156079486,8.37340788319211,-5.37338156945517));
#30985=CARTESIAN_POINT('Ctrl Pts',(19.5746527036711,8.44450649480009,-5.27643569385595));
#30986=CARTESIAN_POINT('Ctrl Pts',(19.6098993308259,8.46026297952948,-5.2549510801074));
#30987=CARTESIAN_POINT('Ctrl Pts',(19.6453331883326,8.4758372773732,-5.23366312269295));
#30988=CARTESIAN_POINT('Ctrl Pts',(19.6809626607781,8.49122942455084,-5.21258698920787));
#30989=CARTESIAN_POINT('Ctrl Pts',(19.7602474117224,8.52548091556979,-5.16568716500225));
#30990=CARTESIAN_POINT('Ctrl Pts',(19.84051379949,8.5588361256642,-5.11984028725031));
#30991=CARTESIAN_POINT('Ctrl Pts',(19.9218515401125,8.59129199482057,-5.0752193141543));
#30992=CARTESIAN_POINT('Ctrl Pts',(20.0625119818507,8.64741916109783,-4.99805457195169));
#30993=CARTESIAN_POINT('Ctrl Pts',(20.2064041971235,8.70084633312459,-4.92460712543744));
#30994=CARTESIAN_POINT('Ctrl Pts',(20.3542553451009,8.75145781928091,-4.85625190593564));
#30995=CARTESIAN_POINT('Ctrl Pts',(20.4095323426498,8.77037989756356,-4.83069599140576));
#30996=CARTESIAN_POINT('Ctrl Pts',(20.4654213730509,8.78892550132495,-4.80583004620885));
#30997=CARTESIAN_POINT('Ctrl Pts',(20.521903888801,8.80706270078843,-4.78177653697074));
#30998=CARTESIAN_POINT('Ctrl Pts',(20.6157677318787,8.83720348367853,-4.74180390496927));
#30999=CARTESIAN_POINT('Ctrl Pts',(20.7113661107907,8.86624663007563,-4.70403416052498));
#31000=CARTESIAN_POINT('Ctrl Pts',(20.8085605831725,8.89401965877196,-4.66907541654005));
#31001=CARTESIAN_POINT('Ctrl Pts',(20.9633493392486,8.93825008113056,-4.61340125768304));
#31002=CARTESIAN_POINT('Ctrl Pts',(21.1207753957801,8.97886804824034,-4.56536356405399));
#31003=CARTESIAN_POINT('Ctrl Pts',(21.2809696644016,9.01563161793901,-4.5267531020893));
#31004=CARTESIAN_POINT('Ctrl Pts',(21.336234501468,9.02831454790188,-4.51343301949271));
#31005=CARTESIAN_POINT('Ctrl Pts',(21.3918288587508,9.04053919558814,-4.50123584390736));
#31006=CARTESIAN_POINT('Ctrl Pts',(21.4477584918535,9.05229263672872,-4.49023354869004));
#31007=CARTESIAN_POINT('Ctrl Pts',(21.5532816474144,9.07446800475902,-4.46947537729971));
#31008=CARTESIAN_POINT('Ctrl Pts',(21.6601522838149,9.09499736369338,-4.45294294540509));
#31009=CARTESIAN_POINT('Ctrl Pts',(21.7683635816266,9.11377672757539,-4.44114927475493));
#31010=CARTESIAN_POINT('Ctrl Pts',(21.8810210295216,9.1333276917614,-4.42887102965826));
#31011=CARTESIAN_POINT('Ctrl Pts',(21.9955129281085,9.15099632977271,-4.42182667462028));
#31012=CARTESIAN_POINT('Ctrl Pts',(22.10992749631,9.16648564567108,-4.42027479233514));
#31013=CARTESIAN_POINT('Ctrl Pts',(22.1631021639207,9.17368437252344,-4.41955354830145));
#31014=CARTESIAN_POINT('Ctrl Pts',(22.2162597933297,9.18041259694753,-4.42001800971797));
#31015=CARTESIAN_POINT('Ctrl Pts',(22.269207906859,9.18664184844023,-4.42169059515386));
#31016=CARTESIAN_POINT('Ctrl Pts',(22.3245959938815,9.1931581584797,-4.42344025725701));
#31017=CARTESIAN_POINT('Ctrl Pts',(22.3798739843465,9.19915414218571,-4.42648583520025));
#31018=CARTESIAN_POINT('Ctrl Pts',(22.4350297409268,9.20463704953186,-4.43079673600685));
#31019=CARTESIAN_POINT('Ctrl Pts',(22.5461903148917,9.21568726741267,-4.43948489908678));
#31020=CARTESIAN_POINT('Ctrl Pts',(22.6568734623399,9.22465589712528,-4.45331387784003));
#31021=CARTESIAN_POINT('Ctrl Pts',(22.7671112483177,9.23161636460099,-4.4720418464562));
#31022=CARTESIAN_POINT('Ctrl Pts',(22.9323771759594,9.24205133573172,-4.50011838190857));
#31023=CARTESIAN_POINT('Ctrl Pts',(23.0966436253579,9.24797370980892,-4.53919106328867));
#31024=CARTESIAN_POINT('Ctrl Pts',(23.2600592455111,9.24956272808001,-4.58811728405156));
#31025=CARTESIAN_POINT('Ctrl Pts',(23.3115335439096,9.25006325306392,-4.60352855798425));
#31026=CARTESIAN_POINT('Ctrl Pts',(23.3626670235205,9.25013116823148,-4.61983815301514));
#31027=CARTESIAN_POINT('Ctrl Pts',(23.4134608761142,9.24978288855012,-4.63697771253073));
#31028=CARTESIAN_POINT('',(30.8496157942439,5.41463414634146,-4.65853571252146));
#31029=CARTESIAN_POINT('Ctrl Pts',(23.4134608743401,9.24978230648852,-4.63697771328011));
#31030=CARTESIAN_POINT('Ctrl Pts',(24.1431288109746,9.24477620324172,-4.63909799546488));
#31031=CARTESIAN_POINT('Ctrl Pts',(24.8609128854776,9.15469739384237,-4.64118229168175));
#31032=CARTESIAN_POINT('Ctrl Pts',(25.9199435996119,8.89326151785136,-4.64425549764083));
#31033=CARTESIAN_POINT('Ctrl Pts',(26.2686099494916,8.78489606818956,-4.64526695104862));
#31034=CARTESIAN_POINT('Ctrl Pts',(26.9440345067492,8.53086155850978,-4.64722569661479));
#31035=CARTESIAN_POINT('Ctrl Pts',(27.2727683495141,8.38474358569576,-4.64817872235552));
#31036=CARTESIAN_POINT('Ctrl Pts',(27.9124127490458,8.05459039487177,-4.65003256384236));
#31037=CARTESIAN_POINT('Ctrl Pts',(28.2233249304724,7.87055863316035,-4.65093338408782));
#31038=CARTESIAN_POINT('Ctrl Pts',(28.8267164809711,7.46328115931847,-4.65268114057206));
#31039=CARTESIAN_POINT('Ctrl Pts',(29.1157096677008,7.24216864268044,-4.65351797766775));
#31040=CARTESIAN_POINT('Ctrl Pts',(29.9348006057639,6.5362496484837,-4.65588924421514));
#31041=CARTESIAN_POINT('Ctrl Pts',(30.4224818233768,6.00624210868884,-4.65730028266099));
#31042=CARTESIAN_POINT('Ctrl Pts',(30.8496157942439,5.41463414634146,-4.65853571252146));
#31043=CARTESIAN_POINT('',(30.8496157942439,5.41463414634146,-3.60555127546399));
#31044=CARTESIAN_POINT('',(30.8496157942439,5.41463414634146,-12.25));
#31045=CARTESIAN_POINT('',(30.4989465761475,5.86984351166101,-2.5869876306867));
#31046=CARTESIAN_POINT('Ctrl Pts',(30.849615794244,5.41463414634146,-3.605551275464));
#31047=CARTESIAN_POINT('Ctrl Pts',(30.7816497053553,5.50877154139453,-3.43196160315339));
#31048=CARTESIAN_POINT('Ctrl Pts',(30.7160583188014,5.59589449756247,-3.25442003177252));
#31049=CARTESIAN_POINT('Ctrl Pts',(30.6537765048508,5.67603715897922,-3.0726189144622));
#31050=CARTESIAN_POINT('Ctrl Pts',(30.5994521176086,5.745940405164,-2.91404558990133));
#31051=CARTESIAN_POINT('Ctrl Pts',(30.547644964311,5.81053321239433,-2.75223195116567));
#31052=CARTESIAN_POINT('Ctrl Pts',(30.4989465761475,5.86984351166102,-2.5869876306867));
#31053=CARTESIAN_POINT('',(29.864460066962,6.56691023510737,-0.418815697553238));
#31054=CARTESIAN_POINT('Ctrl Pts',(30.4989465761475,5.86984351166101,-2.5869876306867));
#31055=CARTESIAN_POINT('Ctrl Pts',(30.4233137302993,5.96195758136262,-2.33034877705622));
#31056=CARTESIAN_POINT('Ctrl Pts',(30.3488530146943,6.04900208546168,-2.07155907215208));
#31057=CARTESIAN_POINT('Ctrl Pts',(30.2763686633504,6.13089490379009,-1.81064777642531));
#31058=CARTESIAN_POINT('Ctrl Pts',(30.2474221995087,6.16359861791162,-1.70645343312763));
#31059=CARTESIAN_POINT('Ctrl Pts',(30.2187907831553,6.19548031299598,-1.60192036444818));
#31060=CARTESIAN_POINT('Ctrl Pts',(30.1905253828516,6.22653294269323,-1.4970490342653));
#31061=CARTESIAN_POINT('Ctrl Pts',(30.1904920035368,6.22656961351661,-1.496925189101));
#31062=CARTESIAN_POINT('Ctrl Pts',(30.1904586247358,6.22660628317995,-1.49680134349088));
#31063=CARTESIAN_POINT('Ctrl Pts',(30.1904252464487,6.22664295168324,-1.49667749743492));
#31064=CARTESIAN_POINT('Ctrl Pts',(30.1409379935327,6.28100833875472,-1.31306109194066));
#31065=CARTESIAN_POINT('Ctrl Pts',(30.0927220038854,6.33270175377753,-1.12832912483359));
#31066=CARTESIAN_POINT('Ctrl Pts',(30.0443718207765,6.38340707955811,-0.943346491560341));
#31067=CARTESIAN_POINT('Ctrl Pts',(30.0441587992402,6.38363047739661,-0.9425314939285));
#31068=CARTESIAN_POINT('Ctrl Pts',(30.043945774759,6.38385385639887,-0.941716493265572));
#31069=CARTESIAN_POINT('Ctrl Pts',(30.043732747184,6.38407721673838,-0.940901489514493));
#31070=CARTESIAN_POINT('Ctrl Pts',(30.0318497332597,6.39653660855655,-0.895439295599127));
#31071=CARTESIAN_POINT('Ctrl Pts',(30.0199872914384,6.40890822298575,-0.849938922706313));
#31072=CARTESIAN_POINT('Ctrl Pts',(30.0079304061828,6.42140928985854,-0.804534650823485));
#31073=CARTESIAN_POINT('Ctrl Pts',(29.9956573763493,6.4341344641823,-0.758316413561679));
#31074=CARTESIAN_POINT('Ctrl Pts',(29.9831839646327,6.44699262206468,-0.712196692305319));
#31075=CARTESIAN_POINT('Ctrl Pts',(29.9702866480314,6.46020934529529,-0.666313906124657));
#31076=CARTESIAN_POINT('Ctrl Pts',(29.9699605773387,6.4605434912446,-0.66515389491177));
#31077=CARTESIAN_POINT('Ctrl Pts',(29.9696342279293,6.46087787433656,-0.663994050439389));
#31078=CARTESIAN_POINT('Ctrl Pts',(29.9693075950715,6.46121249935582,-0.662834372594784));
#31079=CARTESIAN_POINT('Ctrl Pts',(29.9631744517615,6.46749571045688,-0.641059250330851));
#31080=CARTESIAN_POINT('Ctrl Pts',(29.9569646332742,6.47384124142273,-0.619325925282544));
#31081=CARTESIAN_POINT('Ctrl Pts',(29.9504968110584,6.48042900761182,-0.597745652821244));
#31082=CARTESIAN_POINT('Ctrl Pts',(29.9470906715231,6.48389831306226,-0.586380866226969));
#31083=CARTESIAN_POINT('Ctrl Pts',(29.9436136737991,6.48743408574019,-0.575058008090102));
#31084=CARTESIAN_POINT('Ctrl Pts',(29.9400404044472,6.4910615037687,-0.563792529383379));
#31085=CARTESIAN_POINT('Ctrl Pts',(29.9364671350954,6.49468892179722,-0.552527050676656));
#31086=CARTESIAN_POINT('Ctrl Pts',(29.932797593809,6.49840798487454,-0.541318951401599));
#31087=CARTESIAN_POINT('Ctrl Pts',(29.9290063693871,6.50224387307707,-0.530183682526388));
#31088=CARTESIAN_POINT('Ctrl Pts',(29.9286162428098,6.50263859567036,-0.529037835208793));
#31089=CARTESIAN_POINT('Ctrl Pts',(29.9282247857061,6.50303459785586,-0.527892544830234));
#31090=CARTESIAN_POINT('Ctrl Pts',(29.9278319485658,6.50343192910026,-0.526747936182566));
#31091=CARTESIAN_POINT('Ctrl Pts',(29.9263160029589,6.50496521730708,-0.522330929049072));
#31092=CARTESIAN_POINT('Ctrl Pts',(29.9247791427553,6.50651870299062,-0.51791532037233));
#31093=CARTESIAN_POINT('Ctrl Pts',(29.923212672742,6.508100959667,-0.513520375041475));
#31094=CARTESIAN_POINT('Ctrl Pts',(29.9224730227865,6.50884806371013,-0.511445186183043));
#31095=CARTESIAN_POINT('Ctrl Pts',(29.9217268013933,6.50960155180301,-0.509373934703031));
#31096=CARTESIAN_POINT('Ctrl Pts',(29.9209731281652,6.51036229090339,-0.507307791346001));
#31097=CARTESIAN_POINT('Ctrl Pts',(29.9183352718667,6.51302487775473,-0.500076289596397));
#31098=CARTESIAN_POINT('Ctrl Pts',(29.9156061316007,6.51577629047366,-0.492907362352822));
#31099=CARTESIAN_POINT('Ctrl Pts',(29.9127479518585,6.51865369130352,-0.485851205288294));
#31100=CARTESIAN_POINT('Ctrl Pts',(29.9113188619874,6.52009239171845,-0.48232312675603));
#31101=CARTESIAN_POINT('Ctrl Pts',(29.9098575120245,6.52156258893556,-0.478823240768701));
#31102=CARTESIAN_POINT('Ctrl Pts',(29.9083591815029,6.52306892717838,-0.475357821786246));
#31103=CARTESIAN_POINT('Ctrl Pts',(29.9079845988725,6.52344551173908,-0.474491467040632));
#31104=CARTESIAN_POINT('Ctrl Pts',(29.9076077049551,6.52382435511173,-0.473627266482822));
#31105=CARTESIAN_POINT('Ctrl Pts',(29.9072284259906,6.52420552985917,-0.472765318151248));
#31106=CARTESIAN_POINT('Ctrl Pts',(29.9060905890972,6.52534905410146,-0.470179473156526));
#31107=CARTESIAN_POINT('Ctrl Pts',(29.9049312867708,6.52651356070896,-0.467613898198012));
#31108=CARTESIAN_POINT('Ctrl Pts',(29.9037485275245,6.52770100890854,-0.465071240312771));
#31109=CARTESIAN_POINT('Ctrl Pts',(29.9033288342664,6.52812236600652,-0.464168997210231));
#31110=CARTESIAN_POINT('Ctrl Pts',(29.9029063478249,6.52854645079439,-0.463269614505198));
#31111=CARTESIAN_POINT('Ctrl Pts',(29.9024807564583,6.5289735744838,-0.462373498999638));
#31112=CARTESIAN_POINT('Ctrl Pts',(29.9016879290205,6.52976925646165,-0.460704139571641));
#31113=CARTESIAN_POINT('Ctrl Pts',(29.9008844909751,6.53057533159955,-0.459044223607598));
#31114=CARTESIAN_POINT('Ctrl Pts',(29.9000662597657,6.53139594067567,-0.457399865173428));
#31115=CARTESIAN_POINT('Ctrl Pts',(29.8998304861335,6.53163239949107,-0.456926042669205));
#31116=CARTESIAN_POINT('Ctrl Pts',(29.8995935103075,6.53187003887733,-0.45645342429796));
#31117=CARTESIAN_POINT('Ctrl Pts',(29.8993552499751,6.532108940062,-0.455982092705053));
#31118=CARTESIAN_POINT('Ctrl Pts',(29.8992435654444,6.53222092499231,-0.455761156020877));
#31119=CARTESIAN_POINT('Ctrl Pts',(29.8991315986733,6.53233318717316,-0.455540502076082));
#31120=CARTESIAN_POINT('Ctrl Pts',(29.8990193411836,6.53244573497027,-0.455320139382878));
#31121=CARTESIAN_POINT('Ctrl Pts',(29.8989105917404,6.53255476564871,-0.455106663023837));
#31122=CARTESIAN_POINT('Ctrl Pts',(29.8988015694646,6.53266406437131,-0.454893459997586));
#31123=CARTESIAN_POINT('Ctrl Pts',(29.8986922666477,6.53277363874348,-0.454680538042995));
#31124=CARTESIAN_POINT('Ctrl Pts',(29.8969980729862,6.53447204151205,-0.451380247746834));
#31125=CARTESIAN_POINT('Ctrl Pts',(29.8952364806792,6.536236670441,-0.448147484916749));
#31126=CARTESIAN_POINT('Ctrl Pts',(29.8933787760059,6.5380958384941,-0.445011068128653));
#31127=CARTESIAN_POINT('Ctrl Pts',(29.8924499236692,6.53902542252065,-0.443442859734605));
#31128=CARTESIAN_POINT('Ctrl Pts',(29.8914970429738,6.5399786410595,-0.44189873785112));
#31129=CARTESIAN_POINT('Ctrl Pts',(29.8905165433067,6.54095903181656,-0.440382304800807));
#31130=CARTESIAN_POINT('Ctrl Pts',(29.8902714183899,6.54120412950582,-0.440003196538228));
#31131=CARTESIAN_POINT('Ctrl Pts',(29.8900245672838,6.54145092545503,-0.439625818827725));
#31132=CARTESIAN_POINT('Ctrl Pts',(29.8897759338787,6.54169947493436,-0.439250227955585));
#31133=CARTESIAN_POINT('Ctrl Pts',(29.8896826963517,6.54179268098911,-0.439109381378533));
#31134=CARTESIAN_POINT('Ctrl Pts',(29.889589208189,6.54188613363401,-0.438968786075626));
#31135=CARTESIAN_POINT('Ctrl Pts',(29.8894954664315,6.54197983578364,-0.438828445015086));
#31136=CARTESIAN_POINT('Ctrl Pts',(29.8888392741288,6.54263575083105,-0.437846057591307));
#31137=CARTESIAN_POINT('Ctrl Pts',(29.8881706556837,6.54330389161229,-0.436876128043556));
#31138=CARTESIAN_POINT('Ctrl Pts',(29.8874885961489,6.54398525780314,-0.435919674471849));
#31139=CARTESIAN_POINT('Ctrl Pts',(29.8870944326006,6.54437902066664,-0.435366938069227));
#31140=CARTESIAN_POINT('Ctrl Pts',(29.8866948500535,6.54477812955196,-0.434818187012216));
#31141=CARTESIAN_POINT('Ctrl Pts',(29.8862897360135,6.5451826931651,-0.434274045291303));
#31142=CARTESIAN_POINT('Ctrl Pts',(29.8850760327679,6.54639474735693,-0.432643821434411));
#31143=CARTESIAN_POINT('Ctrl Pts',(29.8838119934384,6.54765642037571,-0.431056482531672));
#31144=CARTESIAN_POINT('Ctrl Pts',(29.8824997993162,6.54896534130975,-0.429560752560135));
#31145=CARTESIAN_POINT('Ctrl Pts',(29.8823357196801,6.54912901165925,-0.429373723198144));
#31146=CARTESIAN_POINT('Ctrl Pts',(29.8821708786823,6.5492934291796,-0.429188102306744));
#31147=CARTESIAN_POINT('Ctrl Pts',(29.8820052778696,6.54945859195111,-0.429003977866343));
#31148=CARTESIAN_POINT('Ctrl Pts',(29.8818448520823,6.54961859338601,-0.428825607314705));
#31149=CARTESIAN_POINT('Ctrl Pts',(29.8816837132265,6.54977929422165,-0.428648641147257));
#31150=CARTESIAN_POINT('Ctrl Pts',(29.8815218627084,6.54994069271304,-0.428473159351318));
#31151=CARTESIAN_POINT('Ctrl Pts',(29.8779847464994,6.55346793023428,-0.424638142247988));
#31152=CARTESIAN_POINT('Ctrl Pts',(29.8741093126001,6.55732678218991,-0.421508010922387));
#31153=CARTESIAN_POINT('Ctrl Pts',(29.8699063654193,6.56150301427952,-0.419927508649726));
#31154=CARTESIAN_POINT('Ctrl Pts',(29.8681474715732,6.5632507281113,-0.419266083320906));
#31155=CARTESIAN_POINT('Ctrl Pts',(29.8663314430105,6.56505380581228,-0.418875903796053));
#31156=CARTESIAN_POINT('Ctrl Pts',(29.864460066962,6.56691023510737,-0.418815697553239));
#31157=CARTESIAN_POINT('Ctrl Pts',(29.864460066962,6.56691023510738,-0.418815697553238));
#31158=CARTESIAN_POINT('Ctrl Pts',(29.4803688233762,6.9479337269518,-0.406458645803864));
#31159=CARTESIAN_POINT('Ctrl Pts',(29.0688833692417,7.28992300517486,-0.3927064137635));
#31160=CARTESIAN_POINT('Ctrl Pts',(28.6310287709774,7.59430983868232,-0.377052593566359));
#31161=CARTESIAN_POINT('Ctrl Pts',(28.5761396683459,7.63246752895278,-0.375090243172456));
#31162=CARTESIAN_POINT('Ctrl Pts',(28.5208361379456,7.67003424468116,-0.373098007376688));
#31163=CARTESIAN_POINT('Ctrl Pts',(28.4651201665043,7.70701275996229,-0.371074886541032));
#31164=CARTESIAN_POINT('Ctrl Pts',(28.4648104733999,7.70721830230314,-0.371063641173575));
#31165=CARTESIAN_POINT('Ctrl Pts',(28.4645007674488,7.70742382634658,-0.371052394838906));
#31166=CARTESIAN_POINT('Ctrl Pts',(28.4641910486506,7.70762933209214,-0.371041147536674));
#31167=CARTESIAN_POINT('Ctrl Pts',(28.214388439779,7.87337926936937,-0.361969675425142));
#31168=CARTESIAN_POINT('Ctrl Pts',(27.9562330077088,8.02722271600796,-0.35226895739612));
#31169=CARTESIAN_POINT('Ctrl Pts',(27.6895545622681,8.16889014500123,-0.341754746575349));
#31170=CARTESIAN_POINT('Ctrl Pts',(27.6890674556282,8.16914891036643,-0.341735541641497));
#31171=CARTESIAN_POINT('Ctrl Pts',(27.6885803173177,8.16940763590204,-0.341716333849271));
#31172=CARTESIAN_POINT('Ctrl Pts',(27.6880931473781,8.16966632158906,-0.341697123198757));
#31173=CARTESIAN_POINT('Ctrl Pts',(27.4215277388687,8.31121170489137,-0.331185606609609));
#31174=CARTESIAN_POINT('Ctrl Pts',(27.1454796620243,8.44083288074727,-0.319817779335625));
#31175=CARTESIAN_POINT('Ctrl Pts',(26.8667371201343,8.55541115481146,-0.307607446891298));
#31176=CARTESIAN_POINT('Ctrl Pts',(26.8660732568102,8.55568403857499,-0.307578366321717));
#31177=CARTESIAN_POINT('Ctrl Pts',(26.8654093710373,8.55595684207196,-0.30754928159864));
#31178=CARTESIAN_POINT('Ctrl Pts',(26.8647454628164,8.55622956530339,-0.307520192712224));
#31179=CARTESIAN_POINT('Ctrl Pts',(26.3393506191311,8.77205364316396,-0.284500217281987));
#31180=CARTESIAN_POINT('Ctrl Pts',(25.799870653803,8.93761716527978,-0.25887481178718));
#31181=CARTESIAN_POINT('Ctrl Pts',(25.2467440839775,9.05344973047515,-0.225765235501146));
#31182=CARTESIAN_POINT('Ctrl Pts',(25.2124847851188,9.06062411457651,-0.223714509806617));
#31183=CARTESIAN_POINT('Ctrl Pts',(25.1781731384515,9.06760773287862,-0.221635078942255));
#31184=CARTESIAN_POINT('Ctrl Pts',(25.143809249779,9.0744007171519,-0.219525786381147));
#31185=CARTESIAN_POINT('Ctrl Pts',(25.1428439684928,9.07459153201161,-0.219466536374384));
#31186=CARTESIAN_POINT('Ctrl Pts',(25.1418786392007,9.07478219599054,-0.21940726454339));
#31187=CARTESIAN_POINT('Ctrl Pts',(25.1409132619708,9.07497270906429,-0.219347970745587));
#31188=CARTESIAN_POINT('Ctrl Pts',(24.8468326636315,9.13300825930098,-0.201285440372893));
#31189=CARTESIAN_POINT('Ctrl Pts',(24.5482782341044,9.17704104931834,-0.181185608761272));
#31190=CARTESIAN_POINT('Ctrl Pts',(24.2472922152141,9.20637641423141,-0.155024952944712));
#31191=CARTESIAN_POINT('Ctrl Pts',(24.2462473257163,9.20647825356211,-0.154934134791034));
#31192=CARTESIAN_POINT('Ctrl Pts',(24.2452024316097,9.20657991366609,-0.154843252774193));
#31193=CARTESIAN_POINT('Ctrl Pts',(24.2441575329877,9.20668139455152,-0.154752305929168));
#31194=CARTESIAN_POINT('Ctrl Pts',(24.0941447324839,9.22125068529444,-0.14169535415231));
#31195=CARTESIAN_POINT('Ctrl Pts',(23.9440399212374,9.23212605584461,-0.127301668598929));
#31196=CARTESIAN_POINT('Ctrl Pts',(23.7940966118025,9.2393332118484,-0.108714691115995));
#31197=CARTESIAN_POINT('Ctrl Pts',(23.7930931044887,9.23938144630307,-0.108590296316943));
#31198=CARTESIAN_POINT('Ctrl Pts',(23.7920895941272,9.23942951656461,-0.108465732409656));
#31199=CARTESIAN_POINT('Ctrl Pts',(23.7910860815245,9.23947742263663,-0.108340994413874));
#31200=CARTESIAN_POINT('Ctrl Pts',(23.7165180424478,9.24303718047232,-0.0990720846670683));
#31201=CARTESIAN_POINT('Ctrl Pts',(23.6420034506113,9.24568741560599,-0.0888545330623582));
#31202=CARTESIAN_POINT('Ctrl Pts',(23.5678498899834,9.24743431582237,-0.0756482682786467));
#31203=CARTESIAN_POINT('Ctrl Pts',(23.5669491575255,9.24745553516386,-0.0754878537113851));
#31204=CARTESIAN_POINT('Ctrl Pts',(23.5660485062894,9.24747662022085,-0.0753270522346912));
#31205=CARTESIAN_POINT('Ctrl Pts',(23.5651479404179,9.24749757107011,-0.0751658425171525));
#31206=CARTESIAN_POINT('Ctrl Pts',(23.5284025808081,9.24835241857714,-0.0685880793227154));
#31207=CARTESIAN_POINT('Ctrl Pts',(23.4918351889453,9.2489830059991,-0.0613344717879373));
#31208=CARTESIAN_POINT('Ctrl Pts',(23.4557284619252,9.24939573660609,-0.0519736470563747));
#31209=CARTESIAN_POINT('Ctrl Pts',(23.4549670822659,9.24940443982333,-0.0517762560953804));
#31210=CARTESIAN_POINT('Ctrl Pts',(23.4542058832591,9.24941304616209,-0.0515780514109144));
#31211=CARTESIAN_POINT('Ctrl Pts',(23.4534448814482,9.24942155576376,-0.0513789487714902));
#31212=CARTESIAN_POINT('Ctrl Pts',(23.4356451193329,9.24962059456144,-0.0467219564126235));
#31213=CARTESIAN_POINT('Ctrl Pts',(23.4179889581537,9.24976631161214,-0.0415791200096051));
#31214=CARTESIAN_POINT('Ctrl Pts',(23.4006884106516,9.24986111707689,-0.034896743815993));
#31215=CARTESIAN_POINT('Ctrl Pts',(23.4000808005074,9.24986444672655,-0.0346620530027444));
#31216=CARTESIAN_POINT('Ctrl Pts',(23.3994734618759,9.24986771271723,-0.0344255895231507));
#31217=CARTESIAN_POINT('Ctrl Pts',(23.3988665594379,9.24987091524699,-0.0341871261202171));
#31218=CARTESIAN_POINT('Ctrl Pts',(23.393194545426,9.24990084558269,-0.0319584849449891));
#31219=CARTESIAN_POINT('Ctrl Pts',(23.3875779991193,9.24992512955467,-0.0295571279873106));
#31220=CARTESIAN_POINT('Ctrl Pts',(23.3821729808622,9.24994398093205,-0.026804837660644));
#31221=CARTESIAN_POINT('Ctrl Pts',(23.3794776955015,9.24995338142601,-0.0254323709134002));
#31222=CARTESIAN_POINT('Ctrl Pts',(23.3768348453943,9.24996143411909,-0.0239732602558811));
#31223=CARTESIAN_POINT('Ctrl Pts',(23.3742624517826,9.2499681827706,-0.0224103397596845));
#31224=CARTESIAN_POINT('Ctrl Pts',(23.3738593623926,9.24996924027199,-0.0221654329668209));
#31225=CARTESIAN_POINT('Ctrl Pts',(23.3734522044323,9.24997026479149,-0.021918200656897));
#31226=CARTESIAN_POINT('Ctrl Pts',(23.3730424270331,9.24997125713655,-0.0216682085089925));
#31227=CARTESIAN_POINT('Ctrl Pts',(23.369904732602,9.24997885559263,-0.0197540010101278));
#31228=CARTESIAN_POINT('Ctrl Pts',(23.3666181492267,9.24998457304712,-0.017712833015035));
#31229=CARTESIAN_POINT('Ctrl Pts',(23.3637877463315,9.24998876199755,-0.0153303479388135));
#31230=CARTESIAN_POINT('Ctrl Pts',(23.3598235387692,9.24999462896053,-0.0119934854121405));
#31231=CARTESIAN_POINT('Ctrl Pts',(23.3567454098863,9.24999749331721,-0.00798953227686465));
#31232=CARTESIAN_POINT('Ctrl Pts',(23.3561574375587,9.24999819731105,-0.00274506802632453));
#31233=CARTESIAN_POINT('Ctrl Pts',(23.3560588672729,9.24999831533169,-0.00186586280564814));
#31234=CARTESIAN_POINT('Ctrl Pts',(23.3560304040022,9.24999837253056,-0.000951760491110045));
#31235=CARTESIAN_POINT('Ctrl Pts',(23.3560798277435,9.24999837277875,-1.98299169792971E-9));
#31236=CARTESIAN_POINT('Origin',(31.6603850692973,-6.,-12.25));
#31237=CARTESIAN_POINT('',(31.6603850692973,-5.,-3.60555127546388));
#31238=CARTESIAN_POINT('Origin',(31.6603850692973,-6.,-3.60555127546399));
#31239=CARTESIAN_POINT('',(31.6603850692973,-5.,-4.65853571252147));
#31240=CARTESIAN_POINT('',(31.6603850692973,-5.,-12.25));
#31241=CARTESIAN_POINT('Origin',(31.6603850692973,-6.,-4.65853571252147));
#31242=CARTESIAN_POINT('Origin',(31.6603850692973,6.,-12.25));
#31243=CARTESIAN_POINT('',(31.6603850692973,5.,-4.65853571252146));
#31244=CARTESIAN_POINT('Origin',(31.6603850692973,6.,-4.65853571252146));
#31245=CARTESIAN_POINT('',(31.6603850692973,5.,-3.60555127546399));
#31246=CARTESIAN_POINT('',(31.6603850692973,5.,-12.25));
#31247=CARTESIAN_POINT('Origin',(31.6603850692973,6.,-3.60555127546399));
#31248=CARTESIAN_POINT('Origin',(31.6603850692973,5.,-12.25));
#31249=CARTESIAN_POINT('',(32.1691171325868,5.,-3.60555127546399));
#31250=CARTESIAN_POINT('Origin',(23.3621596556826,5.,0.));
#31251=CARTESIAN_POINT('',(31.6603850692973,5.,-3.60555127546399));
#31252=CARTESIAN_POINT('Origin',(31.6603850692973,-5.,-12.25));
#31253=CARTESIAN_POINT('',(31.6603850692973,-5.,-3.60555127546388));
#31254=CARTESIAN_POINT('Origin',(23.3621596556826,-5.00000000000001,0.));
#31255=CARTESIAN_POINT('Ctrl Pts',(29.9256651987116,6.61722146123576,-0.0297557807112802));
#31256=CARTESIAN_POINT('Ctrl Pts',(29.8674234378362,6.56397053279327,-0.216304525438927));
#31257=CARTESIAN_POINT('Ctrl Pts',(29.864460066962,6.56691023510738,-0.418815697553239));
#31258=CARTESIAN_POINT('Ctrl Pts',(29.4859454402383,7.0470527099288,-0.0278002419024762));
#31259=CARTESIAN_POINT('Ctrl Pts',(29.4356629944171,6.99266939386707,-0.209154663943272));
#31260=CARTESIAN_POINT('Ctrl Pts',(29.432253356123,6.99566489409161,-0.404910666487137));
#31261=CARTESIAN_POINT('Ctrl Pts',(29.0122518974518,7.42509242577045,-0.0257317744209179));
#31262=CARTESIAN_POINT('Ctrl Pts',(28.9691053861043,7.37213789927329,-0.20109030922603));
#31263=CARTESIAN_POINT('Ctrl Pts',(28.9652970371725,7.37504694162835,-0.389236972852743));
#31264=CARTESIAN_POINT('Ctrl Pts',(28.2541034544046,7.91872357544883,-0.0225015885182954));
#31265=CARTESIAN_POINT('Ctrl Pts',(28.2193066048444,7.87034913000682,-0.187059634742587));
#31266=CARTESIAN_POINT('Ctrl Pts',(28.2150317307479,7.87299566940952,-0.36199386194761));
#31267=CARTESIAN_POINT('Ctrl Pts',(27.9927306925325,8.07123684933647,-0.0214007247497678));
#31268=CARTESIAN_POINT('Ctrl Pts',(27.9610163781938,8.02448959484978,-0.182056771104165));
#31269=CARTESIAN_POINT('Ctrl Pts',(27.9565703991337,8.02704348376819,-0.35228226385434));
#31270=CARTESIAN_POINT('Ctrl Pts',(27.4532829707667,8.35132766261088,-0.0191573375898124));
#31271=CARTESIAN_POINT('Ctrl Pts',(27.4273020987592,8.30839838388361,-0.171205631262116));
#31272=CARTESIAN_POINT('Ctrl Pts',(27.4225387252865,8.31073680629592,-0.331227233479106));
#31273=CARTESIAN_POINT('Ctrl Pts',(27.1741459407437,8.4790792417291,-0.0180108315948677));
#31274=CARTESIAN_POINT('Ctrl Pts',(27.1509110455396,8.43840855393471,-0.165335158707994));
#31275=CARTESIAN_POINT('Ctrl Pts',(27.1459961653766,8.44062057060429,-0.319840425193462));
#31276=CARTESIAN_POINT('Ctrl Pts',(26.3281384957242,8.8170194343566,-0.0145767734067967));
#31277=CARTESIAN_POINT('Ctrl Pts',(26.3136110967992,8.78315925951623,-0.146408797766953));
#31278=CARTESIAN_POINT('Ctrl Pts',(26.3082189750152,8.78499234568301,-0.283143105918742));
#31279=CARTESIAN_POINT('Ctrl Pts',(25.7498122714157,8.98393143595614,-0.012298136026498));
#31280=CARTESIAN_POINT('Ctrl Pts',(25.7393784856676,8.95628810851345,-0.13226590849984));
#31281=CARTESIAN_POINT('Ctrl Pts',(25.7337629487011,8.95777986606531,-0.255738121840876));
#31282=CARTESIAN_POINT('Ctrl Pts',(24.8625853761885,9.14937514280772,-0.00875627031697524));
#31283=CARTESIAN_POINT('Ctrl Pts',(24.854581000935,9.13176556219335,-0.104200610475345));
#31284=CARTESIAN_POINT('Ctrl Pts',(24.8488322355087,9.13271117527109,-0.201422710339758));
#31285=CARTESIAN_POINT('Ctrl Pts',(24.5621172854782,9.19032444121584,-0.00755656773431116));
#31286=CARTESIAN_POINT('Ctrl Pts',(24.5551525359009,9.17617850406612,-0.0937897668906999));
#31287=CARTESIAN_POINT('Ctrl Pts',(24.5493473176572,9.17693685209554,-0.18127855553775));
#31288=CARTESIAN_POINT('Ctrl Pts',(24.108465748896,9.22946475773662,-0.00557635783698352));
#31289=CARTESIAN_POINT('Ctrl Pts',(24.102103013715,9.2206234248347,-0.0734246424062645));
#31290=CARTESIAN_POINT('Ctrl Pts',(24.0962646566383,9.22109619601611,-0.14189824629866));
#31291=CARTESIAN_POINT('Ctrl Pts',(23.9570760406083,9.23875711818494,-0.00489255841352439));
#31292=CARTESIAN_POINT('Ctrl Pts',(23.9509623379496,9.2316974291279,-0.0659443870662256));
#31293=CARTESIAN_POINT('Ctrl Pts',(23.9451103869989,9.23207461096955,-0.127435185338512));
#31294=CARTESIAN_POINT('Ctrl Pts',(23.7304221300224,9.24710877356689,-0.00369560630858036));
#31295=CARTESIAN_POINT('Ctrl Pts',(23.7244488524214,9.24272883655924,-0.0514200221845465));
#31296=CARTESIAN_POINT('Ctrl Pts',(23.7185889926675,9.24296254743522,-0.099360999755311));
#31297=CARTESIAN_POINT('Ctrl Pts',(23.6548365752529,9.24896093156313,-0.0032714230986638));
#31298=CARTESIAN_POINT('Ctrl Pts',(23.6489217801125,9.24547672099602,-0.0460828268538334));
#31299=CARTESIAN_POINT('Ctrl Pts',(23.6430586656839,9.24566255860898,-0.0890452900807008));
#31300=CARTESIAN_POINT('Ctrl Pts',(23.5419950086281,9.25035039840065,-0.00249198665734557));
#31301=CARTESIAN_POINT('Ctrl Pts',(23.5361101102027,9.24820589361364,-0.0356850645088389));
#31302=CARTESIAN_POINT('Ctrl Pts',(23.5302452018341,9.24832020150227,-0.068951626680926));
#31303=CARTESIAN_POINT('Ctrl Pts',(23.5045077861791,9.25058086470768,-0.00221154209606147));
#31304=CARTESIAN_POINT('Ctrl Pts',(23.4986354745838,9.24888177359471,-0.0318691204795911));
#31305=CARTESIAN_POINT('Ctrl Pts',(23.4927698292697,9.2489723231015,-0.0615775234007954));
#31306=CARTESIAN_POINT('Ctrl Pts',(23.4489407653687,9.25059023689579,-0.00168033373592259));
#31307=CARTESIAN_POINT('Ctrl Pts',(23.4430734758481,9.24955214356626,-0.0244145411752795));
#31308=CARTESIAN_POINT('Ctrl Pts',(23.4372074649957,9.24960744693854,-0.0471730480279435));
#31309=CARTESIAN_POINT('Ctrl Pts',(23.430512099699,9.2505372510034,-0.00148734722344965));
#31310=CARTESIAN_POINT('Ctrl Pts',(23.4246470785189,9.24971834747212,-0.0216787626321344));
#31311=CARTESIAN_POINT('Ctrl Pts',(23.4187809144113,9.24976197463182,-0.0418867767978843));
#31312=CARTESIAN_POINT('Ctrl Pts',(23.403371063412,9.25038009688579,-0.00111076356707283));
#31313=CARTESIAN_POINT('Ctrl Pts',(23.3975061807919,9.24988429559992,-0.0162555467205808));
#31314=CARTESIAN_POINT('Ctrl Pts',(23.3916399614818,9.24991070032524,-0.0314080342307533));
#31315=CARTESIAN_POINT('Ctrl Pts',(23.3943702298556,9.25031441825653,-0.000971660015808843));
#31316=CARTESIAN_POINT('Ctrl Pts',(23.3885054832099,9.24992551808104,-0.0142418469089325));
#31317=CARTESIAN_POINT('Ctrl Pts',(23.3826392408467,9.24994623900693,-0.0275171890143565));
#31318=CARTESIAN_POINT('Ctrl Pts',(23.3775485047153,9.25016841960209,-0.000613695653578594));
#31319=CARTESIAN_POINT('Ctrl Pts',(23.3716836057147,9.24998029042593,-0.00902103423512527));
#31320=CARTESIAN_POINT('Ctrl Pts',(23.3658173417984,9.24999030033329,-0.0174297620702533));
#31321=CARTESIAN_POINT('Ctrl Pts',(23.3672236677921,9.24999842822739,-0.000399711082514158));
#31322=CARTESIAN_POINT('Ctrl Pts',(23.3613578848224,9.24999839902789,-0.0058628102385145));
#31323=CARTESIAN_POINT('Ctrl Pts',(23.3554916518206,9.24999836982608,-0.0113265471363916));
#31324=CARTESIAN_POINT('Ctrl Pts',(23.3560798278466,9.24999837277863,1.1114590155748E-11));
#31325=CARTESIAN_POINT('Ctrl Pts',(23.3560798278471,9.24999837277875,1.11145901557479E-11));
#31326=CARTESIAN_POINT('Ctrl Pts',(23.3560798278471,9.24999837277875,1.11145901557479E-11));
#31327=CARTESIAN_POINT('Origin',(30.568726020147,7.2768464767406,-0.41881569755326));
#31328=CARTESIAN_POINT('Ctrl Pts',(29.8644600065632,6.56691029503575,-0.418819825507771));
#31329=CARTESIAN_POINT('Ctrl Pts',(29.8647590574648,6.56661351376205,-0.398379188670332));
#31330=CARTESIAN_POINT('Ctrl Pts',(29.8656463748335,6.56691023510728,-0.377955629499233));
#31331=CARTESIAN_POINT('Ctrl Pts',(29.8728343714978,6.55860281663837,-0.419091850166062));
#31332=CARTESIAN_POINT('Ctrl Pts',(29.8782115436644,6.55326768870704,-0.398348099807103));
#31333=CARTESIAN_POINT('Ctrl Pts',(29.884200490205,6.54855448701688,-0.377622540410929));
#31334=CARTESIAN_POINT('Ctrl Pts',(29.8800819130269,6.55138207515269,-0.425969995675749));
#31335=CARTESIAN_POINT('Ctrl Pts',(29.8897499363818,6.54175217037167,-0.404642020874189));
#31336=CARTESIAN_POINT('Ctrl Pts',(29.9002720486976,6.53300459397134,-0.38333825478346));
#31337=CARTESIAN_POINT('Ctrl Pts',(29.8924907668869,6.53899009410551,-0.442589318556842));
#31338=CARTESIAN_POINT('Ctrl Pts',(29.9094054806592,6.52207290338313,-0.419992353306782));
#31339=CARTESIAN_POINT('Ctrl Pts',(29.9277760758933,6.50668389169176,-0.397441088483466));
#31340=CARTESIAN_POINT('Ctrl Pts',(29.8976669478591,6.53380470607085,-0.45228876882253));
#31341=CARTESIAN_POINT('Ctrl Pts',(29.9175524482434,6.51388066947101,-0.429013649275077));
#31342=CARTESIAN_POINT('Ctrl Pts',(29.9392488830213,6.49587018835024,-0.405796768245691));
#31343=CARTESIAN_POINT('Ctrl Pts',(29.9120903594397,6.51932939050281,-0.482562048497315));
#31344=CARTESIAN_POINT('Ctrl Pts',(29.9401818870522,6.49106922804923,-0.457204813104785));
#31345=CARTESIAN_POINT('Ctrl Pts',(29.9712179947108,6.46598442274517,-0.431945103081834));
#31346=CARTESIAN_POINT('Ctrl Pts',(29.9202056092526,6.51114549543016,-0.504588759159602));
#31347=CARTESIAN_POINT('Ctrl Pts',(29.9527979603682,6.47826656633695,-0.477763194146236));
#31348=CARTESIAN_POINT('Ctrl Pts',(29.9892051112283,6.44954244731878,-0.451072033579264));
#31349=CARTESIAN_POINT('Ctrl Pts',(29.9430602275497,6.48802947551604,-0.571085079784156));
#31350=CARTESIAN_POINT('Ctrl Pts',(29.9881729418631,6.44222489898683,-0.539807241634622));
#31351=CARTESIAN_POINT('Ctrl Pts',(30.0398614866482,6.40380994709606,-0.508771304298676));
#31352=CARTESIAN_POINT('Ctrl Pts',(29.956339107267,6.47449825530805,-0.616854862246528));
#31353=CARTESIAN_POINT('Ctrl Pts',(30.0084689143173,6.4213325472565,-0.582474942809098));
#31354=CARTESIAN_POINT('Ctrl Pts',(30.0692934500721,6.3780928359179,-0.548455864922925));
#31355=CARTESIAN_POINT('Ctrl Pts',(29.995208562426,6.4346778775047,-0.754816375285201));
#31356=CARTESIAN_POINT('Ctrl Pts',(30.0675109303063,6.36011843264923,-0.710896214022496));
#31357=CARTESIAN_POINT('Ctrl Pts',(30.1554454871045,6.30433955874164,-0.66767816099171));
#31358=CARTESIAN_POINT('Ctrl Pts',(30.0194181045814,6.40957107285731,-0.847960985155597));
#31359=CARTESIAN_POINT('Ctrl Pts',(30.1036626071983,6.32199819104647,-0.797244914477581));
#31360=CARTESIAN_POINT('Ctrl Pts',(30.2091042861041,6.26062352799595,-0.747681437960539));
#31361=CARTESIAN_POINT('Ctrl Pts',(30.092304518959,6.33314980954348,-1.12681711647389));
#31362=CARTESIAN_POINT('Ctrl Pts',(30.2115890006386,6.20653143108887,-1.0550333875945));
#31363=CARTESIAN_POINT('Ctrl Pts',(30.3706514596258,6.13374391009409,-0.985820942249229));
#31364=CARTESIAN_POINT('Ctrl Pts',(30.1407348577505,6.28123094419676,-1.31242838622513));
#31365=CARTESIAN_POINT('Ctrl Pts',(30.2817692847275,6.12909735050055,-1.22513859180251));
#31366=CARTESIAN_POINT('Ctrl Pts',(30.4779926802797,6.05598466186384,-1.1425333971258));
#31367=CARTESIAN_POINT('Ctrl Pts',(30.2897107926523,6.11757159098365,-1.86523612312724));
#31368=CARTESIAN_POINT('Ctrl Pts',(30.4962880035196,5.88480475057273,-1.72974568641597));
#31369=CARTESIAN_POINT('Ctrl Pts',(30.8081817131166,5.83224880525388,-1.60732611923157));
#31370=CARTESIAN_POINT('Ctrl Pts',(30.3933751772269,5.99841777185359,-2.22895100183562));
#31371=CARTESIAN_POINT('Ctrl Pts',(30.6429929060619,5.70670516719143,-2.05647096278954));
#31372=CARTESIAN_POINT('Ctrl Pts',(31.037876828135,5.69732008134285,-1.910419085916));
#31373=CARTESIAN_POINT('Ctrl Pts',(30.4988949496231,5.86990639476642,-2.58702950046792));
#31374=CARTESIAN_POINT('Ctrl Pts',(30.7855691211664,5.52068951837422,-2.35451845566136));
#31375=CARTESIAN_POINT('Ctrl Pts',(31.2718056654608,5.57521816165486,-2.21741796916003));
#31376=CARTESIAN_POINT('Origin',(31.2718056654608,6.50442118859734,-2.5869876306867));
#31377=CARTESIAN_POINT('Ctrl Pts',(30.4952922544597,5.87429133954168,-2.57456137435286));
#31378=CARTESIAN_POINT('Ctrl Pts',(30.782100878076,5.52542682926995,-2.34331966444516));
#31379=CARTESIAN_POINT('Ctrl Pts',(31.2677682718457,5.57944414885034,-2.20676332755905));
#31380=CARTESIAN_POINT('Ctrl Pts',(30.6026936291125,5.74365115677448,-2.94054961542787));
#31381=CARTESIAN_POINT('Ctrl Pts',(30.8866588414079,5.38513818004545,-2.67536548263577));
#31382=CARTESIAN_POINT('Ctrl Pts',(31.3867827859923,5.45535959932825,-2.5204722442975));
#31383=CARTESIAN_POINT('Ctrl Pts',(30.7245581660918,5.58814855489033,-3.28694957844283));
#31384=CARTESIAN_POINT('Ctrl Pts',(31.0038498616718,5.21939244642611,-2.98485241905066));
#31385=CARTESIAN_POINT('Ctrl Pts',(31.5218261370795,5.30765757528954,-2.81739272720526));
#31386=CARTESIAN_POINT('Ctrl Pts',(30.8540107833037,5.40854159977948,-3.61676245692539));
#31387=CARTESIAN_POINT('Ctrl Pts',(31.12465101472,5.03304526371785,-3.27244402072503));
#31388=CARTESIAN_POINT('Ctrl Pts',(31.6652680269827,5.1370731461929,-3.10007755423114));
#31389=CARTESIAN_POINT('Origin',(31.6603850692973,6.,-3.60555127546399));
#31390=CARTESIAN_POINT('Origin',(31.6603850692973,6.,-3.60555127546399));
#31391=CARTESIAN_POINT('Origin',(31.6603850692973,6.,-3.60555127546399));
#31392=CARTESIAN_POINT('Origin',(-60.4312629272455,6.,-3.60555127546399));
#31393=CARTESIAN_POINT('Origin',(32.1691171325868,6.,-3.60555127546399));
#31394=CARTESIAN_POINT('Origin',(32.1691171325868,6.,-3.60555127546399));
#31395=CARTESIAN_POINT('Origin',(32.1691171325868,6.,-3.60555127546399));
#31396=CARTESIAN_POINT('Origin',(23.3621596556826,6.,0.));
#31397=CARTESIAN_POINT('Origin',(31.6603850692973,6.,-4.65853571252146));
#31398=CARTESIAN_POINT('Origin',(31.6603850692973,6.,-4.65853571252146));
#31399=CARTESIAN_POINT('Origin',(31.6603850692973,6.,-4.65853571252146));
#31400=CARTESIAN_POINT('Ctrl Pts',(30.8533045357049,5.40952138492279,-4.65854638171787));
#31401=CARTESIAN_POINT('Ctrl Pts',(30.8491863429757,5.41523354504457,-9.27174184878108));
#31402=CARTESIAN_POINT('Ctrl Pts',(32.4024604985946,6.5271674864424,-5.07262713991702));
#31403=CARTESIAN_POINT('Ctrl Pts',(30.4152070763528,6.01717418209453,-4.65727924423286));
#31404=CARTESIAN_POINT('Ctrl Pts',(30.4100357196704,6.02337177530084,-9.27185079335277));
#31405=CARTESIAN_POINT('Ctrl Pts',(31.8738489475746,7.26036572944057,-5.07124736770548));
#31406=CARTESIAN_POINT('Ctrl Pts',(29.9132343908611,6.56007337163006,-4.65582684825921));
#31407=CARTESIAN_POINT('Ctrl Pts',(29.9069965319543,6.56635458454684,-9.27197690984398));
#31408=CARTESIAN_POINT('Ctrl Pts',(31.2681650881604,7.91543180449786,-5.06966586821974));
#31409=CARTESIAN_POINT('Ctrl Pts',(29.0687996562968,7.27970396316172,-4.65338215219011));
#31410=CARTESIAN_POINT('Ctrl Pts',(29.0612810766789,7.28562977259251,-9.27219266300731));
#31411=CARTESIAN_POINT('Ctrl Pts',(30.249264051552,8.78374326273839,-5.06700386436201));
#31412=CARTESIAN_POINT('Ctrl Pts',(28.7706261881112,7.5045195286773,-4.6525187043648));
#31413=CARTESIAN_POINT('Ctrl Pts',(28.7626222317122,7.51031058117165,-9.27226941720389));
#31414=CARTESIAN_POINT('Ctrl Pts',(29.8894857961232,9.05500734423689,-5.06606366510161));
#31415=CARTESIAN_POINT('Ctrl Pts',(28.1502182742168,7.91573787763403,-4.65072158676973));
#31416=CARTESIAN_POINT('Ctrl Pts',(28.1413123183606,7.92115484475472,-9.27243052035246));
#31417=CARTESIAN_POINT('Ctrl Pts',(29.1408971363909,9.55118636769414,-5.06410680227826));
#31418=CARTESIAN_POINT('Ctrl Pts',(27.8303931769536,8.10087907780226,-4.64979489842099));
#31419=CARTESIAN_POINT('Ctrl Pts',(27.821054471481,8.10605040905191,-9.272514243178));
#31420=CARTESIAN_POINT('Ctrl Pts',(28.7549938692442,9.77457907404743,-5.06309774114946));
#31421=CARTESIAN_POINT('Ctrl Pts',(27.1720888828603,8.43147682347415,-4.64788686746487));
#31422=CARTESIAN_POINT('Ctrl Pts',(27.1619692903368,8.43607716328527,-9.27268812714177));
#31423=CARTESIAN_POINT('Ctrl Pts',(27.9606791639968,10.1734806965365,-5.06102010612049));
#31424=CARTESIAN_POINT('Ctrl Pts',(26.8336084090208,8.57693065213341,-4.64690552139546));
#31425=CARTESIAN_POINT('Ctrl Pts',(26.8231243399102,8.58119242091901,-9.27277829295943));
#31426=CARTESIAN_POINT('Ctrl Pts',(27.5522661850684,10.3489863345083,-5.05995152857685));
#31427=CARTESIAN_POINT('Ctrl Pts',(26.1377630016309,8.82766358702257,-4.6448874029651));
#31428=CARTESIAN_POINT('Ctrl Pts',(26.126651484303,8.83118310305817,-9.27296539649604));
#31429=CARTESIAN_POINT('Ctrl Pts',(26.7126541019231,10.6515225006985,-5.05775402063852));
#31430=CARTESIAN_POINT('Ctrl Pts',(25.7778982955421,8.93339034065304,-4.64384337398826));
#31431=CARTESIAN_POINT('Ctrl Pts',(25.7665078239556,8.93648699505822,-9.27306302842017));
#31432=CARTESIAN_POINT('Ctrl Pts',(26.2784387542334,10.7790931636271,-5.05661718840979));
#31433=CARTESIAN_POINT('Ctrl Pts',(24.6929742515822,9.18202225043397,-4.64069473154187));
#31434=CARTESIAN_POINT('Ctrl Pts',(24.6806743997377,9.18386771107264,-9.27336026701771));
#31435=CARTESIAN_POINT('Ctrl Pts',(24.9693615852528,11.0790942178401,-5.05318866422855));
#31436=CARTESIAN_POINT('Ctrl Pts',(23.9606020319037,9.25954965162327,-4.63856783364716));
#31437=CARTESIAN_POINT('Ctrl Pts',(23.9480649578887,9.26034679384474,-9.27356456880832));
#31438=CARTESIAN_POINT('Ctrl Pts',(24.0856759871578,11.1726393389832,-5.05087270788839));
#31439=CARTESIAN_POINT('Ctrl Pts',(23.2193295343223,9.24907699337613,-4.63641356863091));
#31440=CARTESIAN_POINT('Ctrl Pts',(23.207169819274,9.2489052015715,-9.27377520050726));
#31441=CARTESIAN_POINT('Ctrl Pts',(23.1912512483198,11.1600029543463,-5.04852695082781));
#31442=CARTESIAN_POINT('Ctrl Pts',(23.3608199269989,11.1532729634477,-5.06590970436805));
#31443=CARTESIAN_POINT('Ctrl Pts',(23.3559710985418,11.138801958104,-5.09636870971951));
#31444=CARTESIAN_POINT('Ctrl Pts',(23.3512201232246,11.1227796717029,-5.12610035313048));
#31445=CARTESIAN_POINT('Ctrl Pts',(23.3465896271706,11.1053240247021,-5.15490162040772));
#31446=CARTESIAN_POINT('Ctrl Pts',(23.3418797587551,11.0875691665787,-5.18419657660481));
#31447=CARTESIAN_POINT('Ctrl Pts',(23.3372945494785,11.0683328667465,-5.21252880312016));
#31448=CARTESIAN_POINT('Ctrl Pts',(23.3328562035503,11.0477509482033,-5.23973798876087));
#31449=CARTESIAN_POINT('Ctrl Pts',(23.3283351879441,11.0267856659916,-5.26745397910974));
#31450=CARTESIAN_POINT('Ctrl Pts',(23.3239665585533,11.0044256733813,-5.29400517632869));
#31451=CARTESIAN_POINT('Ctrl Pts',(23.3197720151725,10.980803455366,-5.31927492433835));
#31452=CARTESIAN_POINT('Ctrl Pts',(23.3154580131966,10.9565084878478,-5.34526434271944));
#31453=CARTESIAN_POINT('Ctrl Pts',(23.3113281462826,10.9308797191587,-5.36989941848476));
#31454=CARTESIAN_POINT('Ctrl Pts',(23.3074042205792,10.9040273043179,-5.39309634457922));
#31455=CARTESIAN_POINT('Ctrl Pts',(23.30346517068,10.8770713907852,-5.41638267982072));
#31456=CARTESIAN_POINT('Ctrl Pts',(23.2997336333505,10.848882976181,-5.43822158177815));
#31457=CARTESIAN_POINT('Ctrl Pts',(23.2962301041906,10.8195249341998,-5.45854814492751));
#31458=CARTESIAN_POINT('Ctrl Pts',(23.2927848639698,10.7906553280341,-5.47853653084243));
#31459=CARTESIAN_POINT('Ctrl Pts',(23.2895600909155,10.760654353199,-5.4970643835706));
#31460=CARTESIAN_POINT('Ctrl Pts',(23.2865740508111,10.7295333552622,-5.51406121620227));
#31461=CARTESIAN_POINT('Ctrl Pts',(23.2852810893787,10.7160578999222,-5.52142087926696));
#31462=CARTESIAN_POINT('Ctrl Pts',(23.2840328739702,10.7023718611015,-5.52849320944327));
#31463=CARTESIAN_POINT('Ctrl Pts',(23.2828308238206,10.6884737128611,-5.53527060182817));
#31464=CARTESIAN_POINT('Ctrl Pts',(23.2796513882161,10.651712960936,-5.55319687774997));
#31465=CARTESIAN_POINT('Ctrl Pts',(23.2768360680739,10.613957098551,-5.56881717513421));
#31466=CARTESIAN_POINT('Ctrl Pts',(23.2743989088803,10.5754946947789,-5.58205636128825));
#31467=CARTESIAN_POINT('Ctrl Pts',(23.2717761315175,10.534102929237,-5.59630386626739));
#31468=CARTESIAN_POINT('Ctrl Pts',(23.2695912980638,10.4918935334026,-5.60779509139924));
#31469=CARTESIAN_POINT('Ctrl Pts',(23.2678586014804,10.4491858295028,-5.61648196879886));
#31470=CARTESIAN_POINT('Ctrl Pts',(23.2658148688682,10.3988116739294,-5.62672822588172));
#31471=CARTESIAN_POINT('Ctrl Pts',(23.2644002050124,10.3477442606575,-5.63307519284311));
#31472=CARTESIAN_POINT('Ctrl Pts',(23.2636332080651,10.2964436468988,-5.63547537799447));
#31473=CARTESIAN_POINT('Ctrl Pts',(23.2627671972425,10.2385204871235,-5.63818541005504));
#31474=CARTESIAN_POINT('Ctrl Pts',(23.2627268559077,10.1802948065651,-5.6358667359521));
#31475=CARTESIAN_POINT('Ctrl Pts',(23.263533211117,10.1223923511815,-5.62843902127006));
#31476=CARTESIAN_POINT('Ctrl Pts',(23.2639716357771,10.0909101160187,-5.62440048682808));
#31477=CARTESIAN_POINT('Ctrl Pts',(23.2646602673992,10.0595233230311,-5.61885097568868));
#31478=CARTESIAN_POINT('Ctrl Pts',(23.2656019440501,10.0283395999061,-5.61177455446721));
#31479=CARTESIAN_POINT('Ctrl Pts',(23.2671983896221,9.9754731338505,-5.59977773866687));
#31480=CARTESIAN_POINT('Ctrl Pts',(23.2695177971326,9.92399532300883,-5.58357606216729));
#31481=CARTESIAN_POINT('Ctrl Pts',(23.2724837537471,9.87434129489678,-5.56346581344797));
#31482=CARTESIAN_POINT('Ctrl Pts',(23.2757491971577,9.8196734625647,-5.54132493692807));
#31483=CARTESIAN_POINT('Ctrl Pts',(23.2797981050074,9.76721027632258,-5.5144435673829));
#31484=CARTESIAN_POINT('Ctrl Pts',(23.2845403622107,9.71751468618776,-5.48319085666352));
#31485=CARTESIAN_POINT('Ctrl Pts',(23.2883092109327,9.6780197466803,-5.45835316148862));
#31486=CARTESIAN_POINT('Ctrl Pts',(23.2925161983746,9.64027247638029,-5.43075214175497));
#31487=CARTESIAN_POINT('Ctrl Pts',(23.2971222524907,9.6045799202608,-5.40059475332545));
#31488=CARTESIAN_POINT('Ctrl Pts',(23.3011856691105,9.57309229070155,-5.37399019544048));
#31489=CARTESIAN_POINT('Ctrl Pts',(23.3055597211743,9.54320452924303,-5.34539527966766));
#31490=CARTESIAN_POINT('Ctrl Pts',(23.3102215256331,9.5151437081236,-5.31498951086506));
#31491=CARTESIAN_POINT('Ctrl Pts',(23.3129951951883,9.49844814615341,-5.29689875738589));
#31492=CARTESIAN_POINT('Ctrl Pts',(23.3158708013444,9.48239961855491,-5.27816776321047));
#31493=CARTESIAN_POINT('Ctrl Pts',(23.3188442014171,9.46704699216216,-5.25884324386485));
#31494=CARTESIAN_POINT('Ctrl Pts',(23.3227492502484,9.44688396186458,-5.23346381632692));
#31495=CARTESIAN_POINT('Ctrl Pts',(23.3267744375398,9.4281134250268,-5.20731048454305));
#31496=CARTESIAN_POINT('Ctrl Pts',(23.3309114958432,9.41068440947216,-5.18040132771481));
#31497=CARTESIAN_POINT('Ctrl Pts',(23.3350828281238,9.3931110010575,-5.15326923861005));
#31498=CARTESIAN_POINT('Ctrl Pts',(23.3393678806161,9.37690163249573,-5.1253670769023));
#31499=CARTESIAN_POINT('Ctrl Pts',(23.3437589204372,9.36205724353143,-5.09671411485491));
#31500=CARTESIAN_POINT('Ctrl Pts',(23.3481443762077,9.34723173205895,-5.06809759055231));
#31501=CARTESIAN_POINT('Ctrl Pts',(23.3526355376376,9.33376849043178,-5.03873076660441));
#31502=CARTESIAN_POINT('Ctrl Pts',(23.35722562536,9.32171392291677,-5.00865683320089));
#31503=CARTESIAN_POINT('Ctrl Pts',(23.3593782227678,9.31606073449098,-4.9945531656887));
#31504=CARTESIAN_POINT('Ctrl Pts',(23.3615525914125,9.31071793545332,-4.98029445988451));
#31505=CARTESIAN_POINT('Ctrl Pts',(23.3637481126768,9.30569287797804,-4.96588820382791));
#31506=CARTESIAN_POINT('Ctrl Pts',(23.3688944674221,9.29391402217532,-4.93211959250706));
#31507=CARTESIAN_POINT('Ctrl Pts',(23.3741025072454,9.28400173534217,-4.89789163347882));
#31508=CARTESIAN_POINT('Ctrl Pts',(23.3793475390172,9.27594399955006,-4.86331291591488));
#31509=CARTESIAN_POINT('Ctrl Pts',(23.3845745401648,9.26791396349586,-4.82885306814737));
#31510=CARTESIAN_POINT('Ctrl Pts',(23.3898383021294,9.26172758375133,-4.79404408151541));
#31511=CARTESIAN_POINT('Ctrl Pts',(23.395115005992,9.2573942639056,-4.75904010029301));
#31512=CARTESIAN_POINT('Ctrl Pts',(23.4003235118704,9.25311694941585,-4.72448852288534));
#31513=CARTESIAN_POINT('Ctrl Pts',(23.4055446650074,9.25064690350392,-4.68974712944241));
#31514=CARTESIAN_POINT('Ctrl Pts',(23.4107557118458,9.24998669647212,-4.65501404155883));
#31515=CARTESIAN_POINT('Ctrl Pts',(23.411657828817,9.24987240389592,-4.64900117907418));
#31516=CARTESIAN_POINT('Ctrl Pts',(23.4125596424264,9.24981229765042,-4.6429886806042));
#31517=CARTESIAN_POINT('Ctrl Pts',(23.4134610336593,9.24980631172449,-4.63697771374339));
#31518=CARTESIAN_POINT('Ctrl Pts',(23.7407619571655,9.2417425355196,-4.76017122167868));
#31519=CARTESIAN_POINT('Ctrl Pts',(22.2581052131567,9.30443264497317,-8.73250381527275));
#31520=CARTESIAN_POINT('Ctrl Pts',(23.66457973822,11.1412914989991,-5.17871622099501));
#31521=CARTESIAN_POINT('Ctrl Pts',(23.5838527574288,9.24837701443423,-4.69515805555824));
#31522=CARTESIAN_POINT('Ctrl Pts',(22.1715287485385,9.28227205649985,-8.80903324352776));
#31523=CARTESIAN_POINT('Ctrl Pts',(23.490707426048,11.1509430734207,-5.10875525275042));
#31524=CARTESIAN_POINT('Ctrl Pts',(23.4236136142519,9.25115309215875,-4.63708387423802));
#31525=CARTESIAN_POINT('Ctrl Pts',(22.1106313281463,9.25892841933612,-8.89170684279919));
#31526=CARTESIAN_POINT('Ctrl Pts',(23.3131450879115,11.1559910950577,-5.04633195118703));
#31527=CARTESIAN_POINT('Ctrl Pts',(23.0965052560008,9.2479723676883,-4.53914929014038));
#31528=CARTESIAN_POINT('Ctrl Pts',(22.0406305439231,9.21636517829358,-9.05096883883774));
#31529=CARTESIAN_POINT('Ctrl Pts',(22.9506736640093,11.1556438435962,-4.94129943123646));
#31530=CARTESIAN_POINT('Ctrl Pts',(22.9322244640352,9.24204169116783,-4.50009212968019));
#31531=CARTESIAN_POINT('Ctrl Pts',(22.0347031030604,9.1981366813795,-9.12437043488707));
#31532=CARTESIAN_POINT('Ctrl Pts',(22.7686327863313,11.1502523788117,-4.89955233099308));
#31533=CARTESIAN_POINT('Ctrl Pts',(22.601998284174,9.22119105391794,-4.44398991580241));
#31534=CARTESIAN_POINT('Ctrl Pts',(22.0626396540039,9.17409017957756,-9.23227690113227));
#31535=CARTESIAN_POINT('Ctrl Pts',(22.4027064790007,11.1286492452038,-4.84001519960698));
#31536=CARTESIAN_POINT('Ctrl Pts',(22.4360515375488,9.2062707034032,-4.42695779702948));
#31537=CARTESIAN_POINT('Ctrl Pts',(22.0969461288735,9.168883245967,-9.26448307520217));
#31538=CARTESIAN_POINT('Ctrl Pts',(22.2188195434826,11.1124371401094,-4.82223930830889));
#31539=CARTESIAN_POINT('Ctrl Pts',(22.1023644694404,9.16701301620337,-4.41641652003192));
#31540=CARTESIAN_POINT('Ctrl Pts',(22.1690030235667,9.17234315197961,-9.26969035127475));
#31541=CARTESIAN_POINT('Ctrl Pts',(21.8490581977948,11.0686622585437,-4.81232681866023));
#31542=CARTESIAN_POINT('Ctrl Pts',(21.9335430214035,9.14244254294621,-4.42314440604185));
#31543=CARTESIAN_POINT('Ctrl Pts',(22.2054462396773,9.18107611879875,-9.24187069747537));
#31544=CARTESIAN_POINT('Ctrl Pts',(21.661985782483,11.0408296166206,-4.82045399638167));
#31545=CARTESIAN_POINT('Ctrl Pts',(21.6031838656795,9.08511086427486,-4.45915125113957));
#31546=CARTESIAN_POINT('Ctrl Pts',(22.2377167051826,9.20360768905055,-9.13809050812787));
#31547=CARTESIAN_POINT('Ctrl Pts',(21.2959121232227,10.9751791255569,-4.86128347077255));
#31548=CARTESIAN_POINT('Ctrl Pts',(21.4408293418957,9.05231840460623,-4.48822269433724));
#31549=CARTESIAN_POINT('Ctrl Pts',(22.2341132638195,9.21686200399614,-9.06491957153717));
#31550=CARTESIAN_POINT('Ctrl Pts',(21.1160057592652,10.9373324408439,-4.89376350993861));
#31551=CARTESIAN_POINT('Ctrl Pts',(21.1211096105402,8.97894474489699,-4.56528168833185));
#31552=CARTESIAN_POINT('Ctrl Pts',(22.1702544220307,9.23658596371069,-8.90266922033884));
#31553=CARTESIAN_POINT('Ctrl Pts',(20.761721732372,10.8521500222688,-4.97937766766415));
#31554=CARTESIAN_POINT('Ctrl Pts',(20.9637426859415,8.93836248783126,-4.61325801902883));
#31555=CARTESIAN_POINT('Ctrl Pts',(22.1126646934585,9.2430926653662,-8.815604632918));
#31556=CARTESIAN_POINT('Ctrl Pts',(20.5873421675309,10.8048130510551,-5.03249953644066));
#31557=CARTESIAN_POINT('Ctrl Pts',(20.6533775196975,8.84967655519081,-4.72488961260549));
#31558=CARTESIAN_POINT('Ctrl Pts',(21.9467029793221,9.24171267207773,-8.65176604079951));
#31559=CARTESIAN_POINT('Ctrl Pts',(20.2434240100882,10.7009666613119,-5.15589424043288));
#31560=CARTESIAN_POINT('Ctrl Pts',(20.5017967315099,8.80196327630676,-4.78803948205891));
#31561=CARTESIAN_POINT('Ctrl Pts',(21.8422688128588,9.23443217585936,-8.5761898974068));
#31562=CARTESIAN_POINT('Ctrl Pts',(20.0754561099999,10.644913701976,-5.22560855463383));
#31563=CARTESIAN_POINT('Ctrl Pts',(20.2067132658722,8.70095212509222,-4.92446247464717));
#31564=CARTESIAN_POINT('Ctrl Pts',(21.6025383820459,9.20382388721751,-8.4499513783311));
#31565=CARTESIAN_POINT('Ctrl Pts',(19.7484717287398,10.5259271136452,-5.37612047005189));
#31566=CARTESIAN_POINT('Ctrl Pts',(20.0627946620671,8.64753209592579,-4.99789368139045));
#31567=CARTESIAN_POINT('Ctrl Pts',(21.4693310632381,9.18140104347433,-8.39815497287525));
#31568=CARTESIAN_POINT('Ctrl Pts',(19.5889943573367,10.4628503478549,-5.45709259294587));
#31569=CARTESIAN_POINT('Ctrl Pts',(19.6399435274182,8.47880310571364,-5.22981959670209));
#31570=CARTESIAN_POINT('Ctrl Pts',(21.0540930964424,9.09375652030717,-8.28451329894513));
#31571=CARTESIAN_POINT('Ctrl Pts',(19.1204295859944,10.2632105486208,-5.71278462460776));
#31572=CARTESIAN_POINT('Ctrl Pts',(19.3697981552916,8.35506889938905,-5.39973069152153));
#31573=CARTESIAN_POINT('Ctrl Pts',(20.7428055844105,9.00839665528852,-8.25231835531753));
#31574=CARTESIAN_POINT('Ctrl Pts',(18.8210793093145,10.1162920672119,-5.9000462023183));
#31575=CARTESIAN_POINT('Ctrl Pts',(18.8465231014693,8.0850404366681,-5.75593885943587));
#31576=CARTESIAN_POINT('Ctrl Pts',(20.1091011680343,8.78661111089581,-8.27115731644347));
#31577=CARTESIAN_POINT('Ctrl Pts',(18.2412339790073,9.79473667310455,-6.29272730255182));
#31578=CARTESIAN_POINT('Ctrl Pts',(18.5933272070726,7.93849035974423,-5.94254947324762));
#31579=CARTESIAN_POINT('Ctrl Pts',(19.7883641219259,8.65484775926693,-8.31467161177097));
#31580=CARTESIAN_POINT('Ctrl Pts',(17.9606655558799,9.61978930542312,-6.49849119520135));
#31581=CARTESIAN_POINT('Ctrl Pts',(18.108340600348,7.62696348416377,-6.31757114103161));
#31582=CARTESIAN_POINT('Ctrl Pts',(19.1687148199052,8.35509365521475,-8.4508622545085));
#31583=CARTESIAN_POINT('Ctrl Pts',(17.4232479642539,9.24709047831589,-6.91219203660589));
#31584=CARTESIAN_POINT('Ctrl Pts',(17.8754091113951,7.46141940260319,-6.5068329586448));
#31585=CARTESIAN_POINT('Ctrl Pts',(18.8667622645576,8.18964072402686,-8.53948871553438));
#31586=CARTESIAN_POINT('Ctrl Pts',(17.1651346929798,9.04866437084577,-7.12106524937581));
#31587=CARTESIAN_POINT('Ctrl Pts',(17.4259063892177,7.10978479208954,-6.88361837145848));
#31588=CARTESIAN_POINT('Ctrl Pts',(18.2867484113725,7.82705740885029,-8.74367560464804));
#31589=CARTESIAN_POINT('Ctrl Pts',(16.6670370817724,8.62645478348271,-7.53711266367819));
#31590=CARTESIAN_POINT('Ctrl Pts',(17.2093611002873,6.92369688326685,-7.0711829314943));
#31591=CARTESIAN_POINT('Ctrl Pts',(18.0064015521297,7.63180988067425,-8.85753153715041));
#31592=CARTESIAN_POINT('Ctrl Pts',(16.4270814913594,8.40267421479281,-7.74433143391629));
#31593=CARTESIAN_POINT('Ctrl Pts',(16.7915601485188,6.52931017355786,-7.44095042941296));
#31594=CARTESIAN_POINT('Ctrl Pts',(17.4699776474557,7.21116075749424,-9.09855744937918));
#31595=CARTESIAN_POINT('Ctrl Pts',(15.9641128692286,7.92771133699107,-8.15307202858187));
#31596=CARTESIAN_POINT('Ctrl Pts',(16.5903133615341,6.32102030483416,-7.62317736202818));
#31597=CARTESIAN_POINT('Ctrl Pts',(17.2117049676949,6.98709902479069,-9.22521672502677));
#31598=CARTESIAN_POINT('Ctrl Pts',(15.7411096725996,7.67653975440558,-8.35462007956716));
#31599=CARTESIAN_POINT('Ctrl Pts',(16.2031446806553,5.87972109786976,-7.9792052599084));
#31600=CARTESIAN_POINT('Ctrl Pts',(16.7193587393204,6.50795989920566,-9.48276769470842));
#31601=CARTESIAN_POINT('Ctrl Pts',(15.3120849184942,7.14371633451588,-8.74861548265883));
#31602=CARTESIAN_POINT('Ctrl Pts',(16.0164899333278,5.64553819281045,-8.15373034271471));
#31603=CARTESIAN_POINT('Ctrl Pts',(16.482150418559,6.25235099264002,-9.61448883029963));
#31604=CARTESIAN_POINT('Ctrl Pts',(15.1052512793004,6.86064228488974,-8.94186563738397));
#31605=CARTESIAN_POINT('Ctrl Pts',(15.4909684360467,4.91507969565495,-8.65057793645775));
#31606=CARTESIAN_POINT('Ctrl Pts',(15.8360790816217,5.47002026758944,-9.98913906363838));
#31607=CARTESIAN_POINT('Ctrl Pts',(14.5229166473954,5.97672576172198,-9.49231103543021));
#31608=CARTESIAN_POINT('Ctrl Pts',(15.1832050299975,4.38890092270191,-8.94897579566626));
#31609=CARTESIAN_POINT('Ctrl Pts',(15.4437153305843,4.88646935114675,-10.2366313764018));
#31610=CARTESIAN_POINT('Ctrl Pts',(14.1818815208225,5.33879252138579,-9.82330325380897));
#31611=CARTESIAN_POINT('Ctrl Pts',(14.7936282028206,3.52847339741587,-9.33030908404118));
#31612=CARTESIAN_POINT('Ctrl Pts',(14.953492875312,3.91856318300104,-10.5580046380276));
#31613=CARTESIAN_POINT('Ctrl Pts',(13.7501882811056,4.29397409879376,-10.2466106841205));
#31614=CARTESIAN_POINT('Ctrl Pts',(14.6754746649165,3.2278437718719,-9.44675123187285));
#31615=CARTESIAN_POINT('Ctrl Pts',(14.8068781272224,3.58487283062697,-10.656336839848));
#31616=CARTESIAN_POINT('Ctrl Pts',(13.6192613872657,3.92866298901994,-10.3759324896199));
#31617=CARTESIAN_POINT('Ctrl Pts',(14.4718580234029,2.61628749337707,-9.6481638527312));
#31618=CARTESIAN_POINT('Ctrl Pts',(14.5564895360256,2.9071846621386,-10.8265016627336));
#31619=CARTESIAN_POINT('Ctrl Pts',(13.3936321360263,3.185098162674,-10.5996927978589));
#31620=CARTESIAN_POINT('Ctrl Pts',(14.3855728281781,2.3039822459725,-9.73393618883941));
#31621=CARTESIAN_POINT('Ctrl Pts',(14.4498967803323,2.55973319778683,-10.9001427667305));
#31622=CARTESIAN_POINT('Ctrl Pts',(13.2980188112511,2.8051729619165,-10.6950206797896));
#31623=CARTESIAN_POINT('Ctrl Pts',(14.2453335983135,1.66563454054454,-9.87363041164593));
#31624=CARTESIAN_POINT('Ctrl Pts',(14.2781912174048,1.8516228470949,-11.0196358705889));
#31625=CARTESIAN_POINT('Ctrl Pts',(13.1426185840695,2.02830937336854,-10.8503077377617));
#31626=CARTESIAN_POINT('Ctrl Pts',(14.1913682276192,1.33959736847006,-9.92756592003646));
#31627=CARTESIAN_POINT('Ctrl Pts',(14.211738551509,1.48849006021389,-11.0663999130354));
#31628=CARTESIAN_POINT('Ctrl Pts',(13.0828191185393,1.63137711985507,-10.910281907528));
#31629=CARTESIAN_POINT('Ctrl Pts',(14.1183867686561,0.672587688372933,-10.0005590742266));
#31630=CARTESIAN_POINT('Ctrl Pts',(14.1226151474584,0.748193939568345,-11.1292768460617));
#31631=CARTESIAN_POINT('Ctrl Pts',(13.0019477730282,0.819164813667982,-10.9914533471288));
#31632=CARTESIAN_POINT('Ctrl Pts',(14.10005646014,0.335334215738292,-10.0189290741656));
#31633=CARTESIAN_POINT('Ctrl Pts',(14.1000688879279,0.372241137368051,-11.1452899367182));
#31634=CARTESIAN_POINT('Ctrl Pts',(12.981635809193,0.408413807466937,-11.0118855214374));
#31635=CARTESIAN_POINT('Ctrl Pts',(14.0999438033074,-0.332212108254802,
-10.019041900077));
#31636=CARTESIAN_POINT('Ctrl Pts',(14.0999314344141,-0.368770536470457,
-11.1453873481658));
#31637=CARTESIAN_POINT('Ctrl Pts',(12.9815109730246,-0.404611297179373,
-11.0120110046255));
#31638=CARTESIAN_POINT('Ctrl Pts',(14.1179004591993,-0.664694731558155,
-10.0010464561665));
#31639=CARTESIAN_POINT('Ctrl Pts',(14.1220155872155,-0.739394626095605,
-11.1297027095952));
#31640=CARTESIAN_POINT('Ctrl Pts',(13.0014088890623,-0.809551999095349,
-10.9919954420619));
#31641=CARTESIAN_POINT('Ctrl Pts',(14.1896347468004,-1.32709812952424,-9.92929871441566));
#31642=CARTESIAN_POINT('Ctrl Pts',(14.2096143866203,-1.47458064058229,-11.0678957127947));
#31643=CARTESIAN_POINT('Ctrl Pts',(13.0808982349024,-1.61615847282446,-10.9122087447037));
#31644=CARTESIAN_POINT('Ctrl Pts',(14.2440819345987,-1.65935479644565,-9.87487858129904));
#31645=CARTESIAN_POINT('Ctrl Pts',(14.2766700735661,-1.84470377647724,-11.0206983934546));
#31646=CARTESIAN_POINT('Ctrl Pts',(13.1412316055102,-2.02066592075089,-10.8516953675167));
#31647=CARTESIAN_POINT('Ctrl Pts',(14.4559527871627,-2.62549667548358,-9.66382702633439));
#31648=CARTESIAN_POINT('Ctrl Pts',(14.5383068586704,-2.92564928123915,-10.838608544174));
#31649=CARTESIAN_POINT('Ctrl Pts',(13.3760074138938,-3.19645531868435,-10.6170855755652));
#31650=CARTESIAN_POINT('Ctrl Pts',(14.6610301802517,-3.23529958684364,-9.46010767782022));
#31651=CARTESIAN_POINT('Ctrl Pts',(14.797274385157,-3.6097730509549,-10.6604338378256));
#31652=CARTESIAN_POINT('Ctrl Pts',(13.6032553377581,-3.9379706819944,-10.3906969750855));
#31653=CARTESIAN_POINT('Ctrl Pts',(15.1843845801438,-4.39182021036076,-8.94781484699701));
#31654=CARTESIAN_POINT('Ctrl Pts',(15.4453374658606,-4.89004382349708,-10.2355491633465));
#31655=CARTESIAN_POINT('Ctrl Pts',(14.1831885897263,-5.34233943366017,-9.82201402046962));
#31656=CARTESIAN_POINT('Ctrl Pts',(15.4928501358146,-4.91768382207714,-8.64879979303374));
#31657=CARTESIAN_POINT('Ctrl Pts',(15.8382253403148,-5.47260629285237,-9.98789683284872));
#31658=CARTESIAN_POINT('Ctrl Pts',(14.5250017742756,-5.97987683694916,-9.49034111898627));
#31659=CARTESIAN_POINT('Ctrl Pts',(16.0154588429638,-5.64411069667211,-8.15470473125201));
#31660=CARTESIAN_POINT('Ctrl Pts',(16.4807916124111,-6.25071253065397,-9.61527551915532));
#31661=CARTESIAN_POINT('Ctrl Pts',(15.1041087196526,-6.8589149628141,-8.94294511605303));
#31662=CARTESIAN_POINT('Ctrl Pts',(16.1997926205015,-5.87571307364266,-7.98231314503237));
#31663=CARTESIAN_POINT('Ctrl Pts',(16.7151650787374,-6.50365717348269,-9.48502957169505));
#31664=CARTESIAN_POINT('Ctrl Pts',(15.3083704732675,-7.13887424906056,-8.75205577992599));
#31665=CARTESIAN_POINT('Ctrl Pts',(16.5885891387386,-6.31923989565411,-7.62473779388686));
#31666=CARTESIAN_POINT('Ctrl Pts',(17.2095626811808,-6.98524577388381,-9.2262661640785));
#31667=CARTESIAN_POINT('Ctrl Pts',(15.7391990475312,-7.67439286523923,-8.35634595037217));
#31668=CARTESIAN_POINT('Ctrl Pts',(16.7921363319381,-6.52995311691278,-7.44041803646221));
#31669=CARTESIAN_POINT('Ctrl Pts',(17.4708015184657,-7.21192656737724,-9.0981285045576));
#31670=CARTESIAN_POINT('Ctrl Pts',(15.9647513427821,-7.92848739989083,-8.15248290996759));
#31671=CARTESIAN_POINT('Ctrl Pts',(17.2121549286183,-6.92623429272213,-7.06873293473742));
#31672=CARTESIAN_POINT('Ctrl Pts',(18.0100906225307,-7.63457381075248,-8.85593723561199));
#31673=CARTESIAN_POINT('Ctrl Pts',(16.4301773551509,-8.40572826049159,-7.74162382709166));
#31674=CARTESIAN_POINT('Ctrl Pts',(17.4293842420214,-7.11268557699717,-6.88063705161154));
#31675=CARTESIAN_POINT('Ctrl Pts',(18.2912497012959,-7.83009389817568,-8.7419225173432));
#31676=CARTESIAN_POINT('Ctrl Pts',(16.6708909186913,-8.62994147543376,-7.53381951966801));
#31677=CARTESIAN_POINT('Ctrl Pts',(17.8792347652403,-7.46422901691747,-6.50369336197627));
#31678=CARTESIAN_POINT('Ctrl Pts',(18.8717133714707,-8.19249183101686,-8.53793037040513));
#31679=CARTESIAN_POINT('Ctrl Pts',(17.1693739309962,-9.05203412564116,-7.11759968080442));
#31680=CARTESIAN_POINT('Ctrl Pts',(18.1118335517547,-7.62931683180686,-6.31480630165245));
#31681=CARTESIAN_POINT('Ctrl Pts',(19.1730958355485,-8.35735093042499,-8.44974107184639));
#31682=CARTESIAN_POINT('Ctrl Pts',(17.4271185320558,-9.24990851491713,-6.9091414254315));
#31683=CARTESIAN_POINT('Ctrl Pts',(18.5948661394437,-7.9393680496501,-5.94142401732326));
#31684=CARTESIAN_POINT('Ctrl Pts',(19.7901868370082,-8.6555775096822,-8.31444537841736));
#31685=CARTESIAN_POINT('Ctrl Pts',(17.9623708592913,-9.62083673142101,-6.49725027823761));
#31686=CARTESIAN_POINT('Ctrl Pts',(18.8452448672861,-8.08433603821065,-5.7568497334406));
#31687=CARTESIAN_POINT('Ctrl Pts',(20.1075342963327,-8.78600595448993,-8.27130268715703));
#31688=CARTESIAN_POINT('Ctrl Pts',(18.239817557234,-9.79389664474636,-6.29373156030851));
#31689=CARTESIAN_POINT('Ctrl Pts',(19.3688604852375,-8.35462962365301,-5.40032841845693));
#31690=CARTESIAN_POINT('Ctrl Pts',(20.7417386093025,-9.00808560232857,-8.25224155607797));
#31691=CARTESIAN_POINT('Ctrl Pts',(18.8200402696357,-10.1157701798982,-5.90070501493886));
#31692=CARTESIAN_POINT('Ctrl Pts',(19.6422136178767,-8.47984841605453,-5.2283819419454));
#31693=CARTESIAN_POINT('Ctrl Pts',(21.0568753448171,-9.09452026307236,-8.28480003990359));
#31694=CARTESIAN_POINT('Ctrl Pts',(19.1229450916605,-10.26445186785,-5.71120023558755));
#31695=CARTESIAN_POINT('Ctrl Pts',(20.0671700727504,-8.64920689557343,-4.99559201149219));
#31696=CARTESIAN_POINT('Ctrl Pts',(21.4735709337441,-9.18219869325014,-8.39957693279326));
#31697=CARTESIAN_POINT('Ctrl Pts',(19.5938427853797,-10.4648296682004,-5.45455476540464));
#31698=CARTESIAN_POINT('Ctrl Pts',(20.2116262715113,-8.70273072020049,-4.92202982910422));
#31699=CARTESIAN_POINT('Ctrl Pts',(21.6069299528932,-9.20451236245352,-8.45183085092374));
#31700=CARTESIAN_POINT('Ctrl Pts',(19.7539158701371,-10.528025719249,-5.37343760461358));
#31701=CARTESIAN_POINT('Ctrl Pts',(20.5073293440887,-8.80375687931068,-4.78564870666182));
#31702=CARTESIAN_POINT('Ctrl Pts',(21.8463416500992,-9.23481277781289,-8.57880710613263));
#31703=CARTESIAN_POINT('Ctrl Pts',(20.0815868428442,-10.6470228590782,-5.22296982983514));
#31704=CARTESIAN_POINT('Ctrl Pts',(20.6587941143368,-8.8513250187248,-4.72274331597064));
#31705=CARTESIAN_POINT('Ctrl Pts',(21.950144168652,-9.24188863040543,-8.65453053690068));
#31706=CARTESIAN_POINT('Ctrl Pts',(20.2494261825329,-10.702901113401,-5.15352385726253));
#31707=CARTESIAN_POINT('Ctrl Pts',(20.9691881873021,-8.93981424967264,-4.61150450922749));
#31708=CARTESIAN_POINT('Ctrl Pts',(22.1149730983979,-9.24295181576889,-8.81857069716009));
#31709=CARTESIAN_POINT('Ctrl Pts',(20.5933763717348,-10.8065086445252,-5.03055909951977));
#31710=CARTESIAN_POINT('Ctrl Pts',(21.1264314986761,-8.98025816049582,-4.56379204973175));
#31711=CARTESIAN_POINT('Ctrl Pts',(22.1718570677214,-9.2363230349133,-8.90552485176888));
#31712=CARTESIAN_POINT('Ctrl Pts',(20.7676189597731,-10.8536794210946,-4.97772638126974));
#31713=CARTESIAN_POINT('Ctrl Pts',(21.4455519698772,-9.05330719736127,-4.48729801630187));
#31714=CARTESIAN_POINT('Ctrl Pts',(22.2344681686058,-9.21650383205574,-9.06712395562859));
#31715=CARTESIAN_POINT('Ctrl Pts',(21.1212389416158,-10.9384756207102,-4.89273232060626));
#31716=CARTESIAN_POINT('Ctrl Pts',(21.6074307679876,-9.08591315593356,-4.4585279467887));
#31717=CARTESIAN_POINT('Ctrl Pts',(22.2375705897678,-9.20328697843773,-9.13973863765263));
#31718=CARTESIAN_POINT('Ctrl Pts',(21.3006181501117,-10.9761020130789,-4.86058352992028));
#31719=CARTESIAN_POINT('Ctrl Pts',(21.9363949761706,-9.14287078778472,-4.42299748379683));
#31720=CARTESIAN_POINT('Ctrl Pts',(22.2048926812382,-9.18091771620324,-9.24242200205805));
#31721=CARTESIAN_POINT('Ctrl Pts',(21.6651460566772,-11.0413157248983,-4.82028039988043));
#31722=CARTESIAN_POINT('Ctrl Pts',(22.1048907604966,-9.16736445942107,-4.41635803485168));
#31723=CARTESIAN_POINT('Ctrl Pts',(22.1684501645743,-9.17223852797182,-9.26999463874004));
#31724=CARTESIAN_POINT('Ctrl Pts',(21.8518576014085,-11.0690591488402,-4.8122511790867));
#31725=CARTESIAN_POINT('Ctrl Pts',(22.4394530739544,-9.206615689037,-4.42720601632188));
#31726=CARTESIAN_POINT('Ctrl Pts',(22.0962240073149,-9.16892796897462,-9.26408083371504));
#31727=CARTESIAN_POINT('Ctrl Pts',(22.2225888135429,-11.1128167238586,-4.82249373339013));
#31728=CARTESIAN_POINT('Ctrl Pts',(22.6053470679695,-9.22145320686374,-4.44443202209375));
#31729=CARTESIAN_POINT('Ctrl Pts',(22.0621296126529,-9.17426072073414,-9.23141868494471));
#31730=CARTESIAN_POINT('Ctrl Pts',(22.4064172934819,-11.1289294582834,-4.84048097506774));
#31731=CARTESIAN_POINT('Ctrl Pts',(22.9345901710377,-9.24213946603061,-4.50062308032295));
#31732=CARTESIAN_POINT('Ctrl Pts',(22.0347284941016,-9.19838211472973,-9.1233615918879));
#31733=CARTESIAN_POINT('Ctrl Pts',(22.771254245437,-11.1503449327046,-4.90011924842924));
#31734=CARTESIAN_POINT('Ctrl Pts',(23.0979412457337,-9.24798849555332,-4.53957417540497));
#31735=CARTESIAN_POINT('Ctrl Pts',(22.0409347063402,-9.21655719993794,-9.05024798954247));
#31736=CARTESIAN_POINT('Ctrl Pts',(22.9522648958751,-11.1556479741126,-4.94175504041852));
#31737=CARTESIAN_POINT('Ctrl Pts',(23.4224245118462,-9.25113936332021,-4.6367329096279));
#31738=CARTESIAN_POINT('Ctrl Pts',(22.1104006734227,-9.25878135062781,-8.89225940304983));
#31739=CARTESIAN_POINT('Ctrl Pts',(23.3118274338947,-11.1559872246472,-5.04595562020784));
#31740=CARTESIAN_POINT('Ctrl Pts',(23.5842228676575,-9.24836752493948,-4.69529858884187));
#31741=CARTESIAN_POINT('Ctrl Pts',(22.1715953285364,-9.28230057369568,-8.80893197595439));
#31742=CARTESIAN_POINT('Ctrl Pts',(23.4911181003785,-11.1509276833783,-5.10890659395469));
#31743=CARTESIAN_POINT('Ctrl Pts',(23.7411245379554,-9.24172719765138,-4.76032146685216));
#31744=CARTESIAN_POINT('Ctrl Pts',(22.2583006396915,-9.30448265446957,-8.73233111548978));
#31745=CARTESIAN_POINT('Ctrl Pts',(23.6649815169331,-11.1412691878794,-5.17887790068865));
#31746=CARTESIAN_POINT('Ctrl Pts',(23.3608103941008,-11.1532440216953,-5.06593335958171));
#31747=CARTESIAN_POINT('Ctrl Pts',(23.3559722305032,-11.138804320256,-5.09632894678172));
#31748=CARTESIAN_POINT('Ctrl Pts',(23.3512065153187,-11.1228190011423,-5.12599866299092));
#31749=CARTESIAN_POINT('Ctrl Pts',(23.3465578204016,-11.1054052152928,-5.15474249120358));
#31750=CARTESIAN_POINT('Ctrl Pts',(23.3418303981347,-11.0876965206065,-5.18397310666727));
#31751=CARTESIAN_POINT('Ctrl Pts',(23.337224112825,-11.0685120446219,-5.21224603668186));
#31752=CARTESIAN_POINT('Ctrl Pts',(23.3327737836655,-11.047987014281,-5.23940280567959));
#31753=CARTESIAN_POINT('Ctrl Pts',(23.3282422691374,-11.0270875549723,-5.26705498349359));
#31754=CARTESIAN_POINT('Ctrl Pts',(23.3238723870196,-11.0047996898859,-5.29355036578414));
#31755=CARTESIAN_POINT('Ctrl Pts',(23.3196880352788,-10.9812554009882,-5.31877288978583));
#31756=CARTESIAN_POINT('Ctrl Pts',(23.315387879271,-10.9570595107707,-5.34469346119934));
#31757=CARTESIAN_POINT('Ctrl Pts',(23.311283395679,-10.9315380356051,-5.36927083384139));
#31758=CARTESIAN_POINT('Ctrl Pts',(23.3073895706749,-10.9048005533827,-5.39242091162555));
#31759=CARTESIAN_POINT('Ctrl Pts',(23.3034822287278,-10.8779702552219,-5.4156513521072));
#31760=CARTESIAN_POINT('Ctrl Pts',(23.2997865168957,-10.8499161036061,-5.43744630453823));
#31761=CARTESIAN_POINT('Ctrl Pts',(23.2963126014671,-10.8207004597727,-5.45774050941342));
#31762=CARTESIAN_POINT('Ctrl Pts',(23.2928965023705,-10.7919710515426,-5.47769695808488));
#31763=CARTESIAN_POINT('Ctrl Pts',(23.289694322584,-10.7621181834791,-5.49620400088566));
#31764=CARTESIAN_POINT('Ctrl Pts',(23.286718800121,-10.7311525663159,-5.51319208968022));
#31765=CARTESIAN_POINT('Ctrl Pts',(23.2853739925347,-10.7171574453269,-5.52086997179056));
#31766=CARTESIAN_POINT('Ctrl Pts',(23.2840755758007,-10.7029343921086,-5.5282373181478));
#31767=CARTESIAN_POINT('Ctrl Pts',(23.2828254101566,-10.6884815434047,-5.53528569817435));
#31768=CARTESIAN_POINT('Ctrl Pts',(23.279658478254,-10.6518694449539,-5.55314072376397));
#31769=CARTESIAN_POINT('Ctrl Pts',(23.276837945852,-10.6142687495006,-5.5687056045139));
#31770=CARTESIAN_POINT('Ctrl Pts',(23.2743937471177,-10.5759656011028,-5.58190860303003));
#31771=CARTESIAN_POINT('Ctrl Pts',(23.2717710871026,-10.53486577794,-5.5960756082745));
#31772=CARTESIAN_POINT('Ctrl Pts',(23.2695814696403,-10.4929578204317,-5.60752453362935));
#31773=CARTESIAN_POINT('Ctrl Pts',(23.2678450316622,-10.4505558414619,-5.61620955990059));
#31774=CARTESIAN_POINT('Ctrl Pts',(23.2657327548319,-10.3989762752072,-5.62677439434617));
#31775=CARTESIAN_POINT('Ctrl Pts',(23.2642908067166,-10.3466661130416,-5.63325169235027));
#31776=CARTESIAN_POINT('Ctrl Pts',(23.2635352842541,-10.2941199808551,-5.63559065520854));
#31777=CARTESIAN_POINT('Ctrl Pts',(23.2627150161734,-10.2370708299206,-5.63813005895872));
#31778=CARTESIAN_POINT('Ctrl Pts',(23.2627034573345,-10.1797382740423,-5.63579433971693));
#31779=CARTESIAN_POINT('Ctrl Pts',(23.2635073144818,-10.1227172982536,-5.62850315363752));
#31780=CARTESIAN_POINT('Ctrl Pts',(23.2639526948926,-10.091124588397,-5.62446344152928));
#31781=CARTESIAN_POINT('Ctrl Pts',(23.264648241806,-10.0596273344297,-5.61890183621911));
#31782=CARTESIAN_POINT('Ctrl Pts',(23.265593203137,-10.0283334039203,-5.61180069629684));
#31783=CARTESIAN_POINT('Ctrl Pts',(23.2671319225926,-9.97737620796019,-5.6002376176848));
#31784=CARTESIAN_POINT('Ctrl Pts',(23.2692956663857,-9.92770792626252,-5.58475854587693));
#31785=CARTESIAN_POINT('Ctrl Pts',(23.2720642636561,-9.87971988451815,-5.56563891702826));
#31786=CARTESIAN_POINT('Ctrl Pts',(23.2751704015229,-9.82588125828915,-5.54418826987111));
#31787=CARTESIAN_POINT('Ctrl Pts',(23.2790386770644,-9.77415227312768,-5.5181532747369));
#31788=CARTESIAN_POINT('Ctrl Pts',(23.2836179425702,-9.72506586357993,-5.48789049047839));
#31789=CARTESIAN_POINT('Ctrl Pts',(23.2873494782671,-9.68506650358983,-5.46323005976016));
#31790=CARTESIAN_POINT('Ctrl Pts',(23.2915531940299,-9.64682123564115,-5.43575978462185));
#31791=CARTESIAN_POINT('Ctrl Pts',(23.2961824949623,-9.61064170173483,-5.40568734159021));
#31792=CARTESIAN_POINT('Ctrl Pts',(23.3002576043707,-9.5787933597996,-5.37921498705466));
#31793=CARTESIAN_POINT('Ctrl Pts',(23.3046625412563,-9.54854647437181,-5.35072529360372));
#31794=CARTESIAN_POINT('Ctrl Pts',(23.3093483241437,-9.52013037227305,-5.32039252488423));
#31795=CARTESIAN_POINT('Ctrl Pts',(23.312399140962,-9.50162923291665,-5.30064348333047));
#31796=CARTESIAN_POINT('Ctrl Pts',(23.3155686554131,-9.48390454945879,-5.28011386077589));
#31797=CARTESIAN_POINT('Ctrl Pts',(23.3188386447889,-9.46702123153851,-5.25886285488616));
#31798=CARTESIAN_POINT('Ctrl Pts',(23.3227566922586,-9.44679191778429,-5.23340024926764));
#31799=CARTESIAN_POINT('Ctrl Pts',(23.3267923117017,-9.42796376054304,-5.20715758246077));
#31800=CARTESIAN_POINT('Ctrl Pts',(23.330940453435,-9.41048602013606,-5.18015433854917));
#31801=CARTESIAN_POINT('Ctrl Pts',(23.3351228528353,-9.39286393880524,-5.15292808679546));
#31802=CARTESIAN_POINT('Ctrl Pts',(23.3394201598385,-9.37661484871459,-5.12492704450796));
#31803=CARTESIAN_POINT('Ctrl Pts',(23.3438276432082,-9.36173991954695,-5.09617140010087));
#31804=CARTESIAN_POINT('Ctrl Pts',(23.3482277973286,-9.34688972605164,-5.06746357374989));
#31805=CARTESIAN_POINT('Ctrl Pts',(23.3527381839121,-9.3334098734431,-5.03800229552381));
#31806=CARTESIAN_POINT('Ctrl Pts',(23.3573474234541,-9.32134719718139,-5.00783018426007));
#31807=CARTESIAN_POINT('Ctrl Pts',(23.3594602261015,-9.31581785679728,-4.99399976473583));
#31808=CARTESIAN_POINT('Ctrl Pts',(23.36159366775,-9.31058685109039,-4.98002042570589));
#31809=CARTESIAN_POINT('Ctrl Pts',(23.3637458539898,-9.3056610997891,-4.9658989442033));
#31810=CARTESIAN_POINT('Ctrl Pts',(23.3689327974921,-9.2937896393951,-4.93186502772874));
#31811=CARTESIAN_POINT('Ctrl Pts',(23.3741744881082,-9.28381406376272,-4.89736287705005));
#31812=CARTESIAN_POINT('Ctrl Pts',(23.3794567597349,-9.27572244423294,-4.86250693594901));
#31813=CARTESIAN_POINT('Ctrl Pts',(23.3847141593254,-9.26766892479876,-4.82781511708374));
#31814=CARTESIAN_POINT('Ctrl Pts',(23.3900119424402,-9.261483515081,-4.79277205245652));
#31815=CARTESIAN_POINT('Ctrl Pts',(23.3953264024608,-9.25717549603294,-4.75753613869458));
#31816=CARTESIAN_POINT('Ctrl Pts',(23.4005606407812,-9.25293250647258,-4.72283211056155));
#31817=CARTESIAN_POINT('Ctrl Pts',(23.4058109474606,-9.25051245822955,-4.68794116925394));
#31818=CARTESIAN_POINT('Ctrl Pts',(23.4110447433103,-9.24991730685651,-4.65306327354699));
#31819=CARTESIAN_POINT('Ctrl Pts',(23.4118483764353,-9.24982592320849,-4.64770788080257));
#31820=CARTESIAN_POINT('Ctrl Pts',(23.4126516036639,-9.24977752137499,-4.64235288481083));
#31821=CARTESIAN_POINT('Ctrl Pts',(23.4134542901992,-9.24977205331206,-4.63699910361382));
#31822=CARTESIAN_POINT('Ctrl Pts',(32.4024604985347,-6.5271674865253,-5.07262713991703));
#31823=CARTESIAN_POINT('Ctrl Pts',(30.8491863429263,-5.4152335451132,-9.27174184877918));
#31824=CARTESIAN_POINT('Ctrl Pts',(30.8533045356553,-5.40952138499152,-4.65854638171772));
#31825=CARTESIAN_POINT('Ctrl Pts',(31.8738489475283,-7.26036572948979,-5.07124736770671));
#31826=CARTESIAN_POINT('Ctrl Pts',(30.4100357196107,-6.02337177536106,-9.27185079334058));
#31827=CARTESIAN_POINT('Ctrl Pts',(30.4152070763148,-6.01717418213576,-4.65727924423418));
#31828=CARTESIAN_POINT('Ctrl Pts',(31.2681650881339,-7.91543180451874,-5.06966586822249));
#31829=CARTESIAN_POINT('Ctrl Pts',(29.9069965319627,-6.56635458453651,-9.27197690985764));
#31830=CARTESIAN_POINT('Ctrl Pts',(29.9132343908402,-6.56007337164787,-4.65582684826234));
#31831=CARTESIAN_POINT('Ctrl Pts',(30.2492640515523,-8.7837432627388,-5.06700386436085));
#31832=CARTESIAN_POINT('Ctrl Pts',(29.061281076665,-7.28562977260592,-9.2721926629975));
#31833=CARTESIAN_POINT('Ctrl Pts',(29.0687996562966,-7.27970396316187,-4.65338215218851));
#31834=CARTESIAN_POINT('Ctrl Pts',(29.8894857961231,-9.05500734423673,-5.06606366510207));
#31835=CARTESIAN_POINT('Ctrl Pts',(28.7626222317253,-7.51031058116255,-9.27226941720439));
#31836=CARTESIAN_POINT('Ctrl Pts',(28.7706261881107,-7.50451952867758,-4.65251870436497));
#31837=CARTESIAN_POINT('Ctrl Pts',(29.1408971363909,-9.55118636769419,-5.06410680227813));
#31838=CARTESIAN_POINT('Ctrl Pts',(28.141312318348,-7.92115484476349,-9.27243052034795));
#31839=CARTESIAN_POINT('Ctrl Pts',(28.1502182742173,-7.91573787763376,-4.65072158676955));
#31840=CARTESIAN_POINT('Ctrl Pts',(28.7549938692441,-9.77457907404737,-5.06309774114963));
#31841=CARTESIAN_POINT('Ctrl Pts',(27.8210544714496,-8.10605040906689,-9.27251424317563));
#31842=CARTESIAN_POINT('Ctrl Pts',(27.830393176953,-8.10087907780255,-4.64979489842099));
#31843=CARTESIAN_POINT('Ctrl Pts',(27.9606791639968,-10.1734806965365,-5.06102010612066));
#31844=CARTESIAN_POINT('Ctrl Pts',(27.1619692903677,-8.43607716327051,-9.2726881271401));
#31845=CARTESIAN_POINT('Ctrl Pts',(27.1720888828609,-8.43147682347387,-4.64788686746487));
#31846=CARTESIAN_POINT('Ctrl Pts',(27.5522661850697,-10.3489863345078,-5.05995152857696));
#31847=CARTESIAN_POINT('Ctrl Pts',(26.8231243399103,-8.58119242091901,-9.27277829295598));
#31848=CARTESIAN_POINT('Ctrl Pts',(26.8336084090221,-8.57693065213295,-4.64690552139547));
#31849=CARTESIAN_POINT('Ctrl Pts',(26.7126541019217,-10.6515225006989,-5.05775402063874));
#31850=CARTESIAN_POINT('Ctrl Pts',(26.126651484303,-8.83118310305816,-9.27296539649543));
#31851=CARTESIAN_POINT('Ctrl Pts',(26.1377630016296,-8.82766358702302,-4.6448874029651));
#31852=CARTESIAN_POINT('Ctrl Pts',(26.2784387542335,-10.7790931636274,-5.05661718840921));
#31853=CARTESIAN_POINT('Ctrl Pts',(25.7665078239556,-8.93648699505751,-9.27306302841706));
#31854=CARTESIAN_POINT('Ctrl Pts',(25.7778982955421,-8.93339034065304,-4.64384337398737));
#31855=CARTESIAN_POINT('Ctrl Pts',(24.9693615852526,-11.0790942178393,-5.05318866423019));
#31856=CARTESIAN_POINT('Ctrl Pts',(24.6806743997377,-9.18386771107407,-9.27336026701782));
#31857=CARTESIAN_POINT('Ctrl Pts',(24.6929742515822,-9.18202225043396,-4.64069473154366));
#31858=CARTESIAN_POINT('Ctrl Pts',(24.0856759871579,-11.1726393389836,-5.05087270788765));
#31859=CARTESIAN_POINT('Ctrl Pts',(23.9480649578886,-9.26034679384409,-9.27356456879131));
#31860=CARTESIAN_POINT('Ctrl Pts',(23.9606020319037,-9.25954965162327,-4.63856783364609));
#31861=CARTESIAN_POINT('Ctrl Pts',(23.1912512483198,-11.1600029543462,-5.04852695082798));
#31862=CARTESIAN_POINT('Ctrl Pts',(23.2071698192741,-9.2489052015715,-9.27377520050524));
#31863=CARTESIAN_POINT('Ctrl Pts',(23.2193295343223,-9.24907699337613,-4.63641356863091));
#31864=CARTESIAN_POINT('Origin',(31.6603850692973,-6.,-4.65853571252147));
#31865=CARTESIAN_POINT('Origin',(31.6603850692973,-6.,-4.65853571252147));
#31866=CARTESIAN_POINT('Origin',(31.6603850692973,-6.,-4.65853571252147));
#31867=CARTESIAN_POINT('Origin',(23.3621596556826,-6.00000000000001,0.));
#31868=CARTESIAN_POINT('Origin',(-60.4312629272455,-6.00000000000007,-3.60555127546388));
#31869=CARTESIAN_POINT('Origin',(31.6603850692973,-6.00000000000007,-3.60555127546388));
#31870=CARTESIAN_POINT('Origin',(31.6603850692973,-6.,-3.60555127546399));
#31871=CARTESIAN_POINT('Origin',(31.6603850692973,-6.,-3.60555127546399));
#31872=CARTESIAN_POINT('Ctrl Pts',(30.8540107833128,-5.40854159976692,-3.61676245694848));
#31873=CARTESIAN_POINT('Ctrl Pts',(31.1246510147285,-5.03304526370463,-3.27244402074537));
#31874=CARTESIAN_POINT('Ctrl Pts',(31.6652680269928,-5.13707314618097,-3.10007755425091));
#31875=CARTESIAN_POINT('Ctrl Pts',(30.7245581660947,-5.58814855488697,-3.28694957845087));
#31876=CARTESIAN_POINT('Ctrl Pts',(31.0038498616761,-5.2193924464231,-2.98485241905846));
#31877=CARTESIAN_POINT('Ctrl Pts',(31.521826137082,-5.3076575752865,-2.81739272721273));
#31878=CARTESIAN_POINT('Ctrl Pts',(30.6026936291093,-5.74365115677863,-2.94054961542029));
#31879=CARTESIAN_POINT('Ctrl Pts',(30.8866588414047,-5.38513818005051,-2.67536548262944));
#31880=CARTESIAN_POINT('Ctrl Pts',(31.3867827859884,-5.45535959933227,-2.52047224429094));
#31881=CARTESIAN_POINT('Ctrl Pts',(30.4952922544521,-5.87429133955086,-2.57456137432713));
#31882=CARTESIAN_POINT('Ctrl Pts',(30.7821008780688,-5.52542682927969,-2.343319664422));
#31883=CARTESIAN_POINT('Ctrl Pts',(31.2677682718374,-5.57944414885907,-2.206763327537));
#31884=CARTESIAN_POINT('Origin',(31.2718056654608,-6.50442118859734,-2.5869876306867));
#31885=CARTESIAN_POINT('Ctrl Pts',(30.5324890548671,-5.82879633920879,-2.71722364618277));
#31886=CARTESIAN_POINT('Ctrl Pts',(30.8338107320096,-5.45071871851039,-2.46481580902341));
#31887=CARTESIAN_POINT('Ctrl Pts',(31.3550349630983,-5.53239849610685,-2.3266043417601));
#31888=CARTESIAN_POINT('Ctrl Pts',(30.414072865639,-5.97470345390586,-2.316286616319));
#31889=CARTESIAN_POINT('Ctrl Pts',(30.6750363657221,-5.66357496609264,-2.13638111093782));
#31890=CARTESIAN_POINT('Ctrl Pts',(31.0916380800151,-5.66597009492328,-1.98109641144098));
#31891=CARTESIAN_POINT('Ctrl Pts',(30.2983091365626,-6.10823981714543,-1.91022886595462));
#31892=CARTESIAN_POINT('Ctrl Pts',(30.5109747166508,-5.86560552736745,-1.77125969601649));
#31893=CARTESIAN_POINT('Ctrl Pts',(30.8338791248953,-5.81481785500372,-1.64351567473586));
#31894=CARTESIAN_POINT('Ctrl Pts',(30.1385677084671,-6.28357646880036,-1.3132741814918));
#31895=CARTESIAN_POINT('Ctrl Pts',(30.2801036148756,-6.12983921074557,-1.22538124018223));
#31896=CARTESIAN_POINT('Ctrl Pts',(30.4777418384395,-6.05616287591927,-1.14217293852664));
#31897=CARTESIAN_POINT('Ctrl Pts',(30.0904315385969,-6.33514385852499,-1.12739899919828));
#31898=CARTESIAN_POINT('Ctrl Pts',(30.2102025602331,-6.20727944608654,-1.05512647412131));
#31899=CARTESIAN_POINT('Ctrl Pts',(30.3703800811856,-6.1339441904561,-0.985420405775108));
#31900=CARTESIAN_POINT('Ctrl Pts',(30.018023994589,-6.41102310169597,-0.848150890259438));
#31901=CARTESIAN_POINT('Ctrl Pts',(30.1026491762848,-6.32269295519541,-0.797099276114036));
#31902=CARTESIAN_POINT('Ctrl Pts',(30.2087777149437,-6.26088647609721,-0.747200281085206));
#31903=CARTESIAN_POINT('Ctrl Pts',(29.9939866367595,-6.43594024923508,-0.754898211424712));
#31904=CARTESIAN_POINT('Ctrl Pts',(30.0666264056926,-6.36077277190929,-0.710692186109099));
#31905=CARTESIAN_POINT('Ctrl Pts',(30.1551143502848,-6.30461258601909,-0.667187369252594));
#31906=CARTESIAN_POINT('Ctrl Pts',(29.9553790818645,-6.47547849065892,-0.616730145059731));
#31907=CARTESIAN_POINT('Ctrl Pts',(30.0077313439108,-6.42194755412475,-0.582137175444621));
#31908=CARTESIAN_POINT('Ctrl Pts',(30.0688833690653,-6.37844917842461,-0.547904805602633));
#31909=CARTESIAN_POINT('Ctrl Pts',(29.9421730778576,-6.48893120155848,-0.570837627283043));
#31910=CARTESIAN_POINT('Ctrl Pts',(29.9874546393352,-6.44285275085176,-0.539374301820755));
#31911=CARTESIAN_POINT('Ctrl Pts',(30.0393820383596,-6.40423350461356,-0.508152377116182));
#31912=CARTESIAN_POINT('Ctrl Pts',(29.9194851596862,-6.51187275945457,-0.504345210892826));
#31913=CARTESIAN_POINT('Ctrl Pts',(29.9521600875081,-6.47885302842194,-0.477362421809093));
#31914=CARTESIAN_POINT('Ctrl Pts',(29.9886822113593,-6.45001927031411,-0.45051366532455));
#31915=CARTESIAN_POINT('Ctrl Pts',(29.9114793064789,-6.51994455052701,-0.482456574337637));
#31916=CARTESIAN_POINT('Ctrl Pts',(29.9396491544529,-6.4915613908261,-0.456942353896258));
#31917=CARTESIAN_POINT('Ctrl Pts',(29.9707897557899,-6.46637912941077,-0.431525520814346));
#31918=CARTESIAN_POINT('Ctrl Pts',(29.8743743869234,-6.55717647646013,-0.404137800076886));
#31919=CARTESIAN_POINT('Ctrl Pts',(29.8811504343294,-6.55057084913525,-0.384098298935905));
#31920=CARTESIAN_POINT('Ctrl Pts',(29.8878444644056,-6.54394119315548,-0.363954837557253));
#31921=CARTESIAN_POINT('Ctrl Pts',(29.8326596614655,-6.59883470986062,-0.326319010490884));
#31922=CARTESIAN_POINT('Ctrl Pts',(29.8141830203482,-6.61768161165595,-0.311268651041244));
#31923=CARTESIAN_POINT('Ctrl Pts',(29.7933669799477,-6.63390835381247,-0.296165474079821));
#31924=CARTESIAN_POINT('Ctrl Pts',(29.6859854969601,-6.74216993980689,-0.814345382263683));
#31925=CARTESIAN_POINT('Ctrl Pts',(29.5721084772451,-6.8527104879045,-0.782222273536295));
#31926=CARTESIAN_POINT('Ctrl Pts',(29.4730487580193,-6.97593588682555,-0.747368780897885));
#31927=CARTESIAN_POINT('Origin',(30.5687260201471,-7.27684647674051,-0.418815697553272));
#31928=CARTESIAN_POINT('Ctrl Pts',(29.8644600669621,-6.56691023510729,-0.418815697553251));
#31929=CARTESIAN_POINT('Ctrl Pts',(29.8672867891358,-6.56410609007334,-0.22564283964309));
#31930=CARTESIAN_POINT('Ctrl Pts',(29.9206004593126,-6.61260230756601,-0.0463738348445692));
#31931=CARTESIAN_POINT('Ctrl Pts',(29.4322533561227,-6.99566489409189,-0.404910666486995));
#31932=CARTESIAN_POINT('Ctrl Pts',(29.4355057872863,-6.99280750543929,-0.218180296639813));
#31933=CARTESIAN_POINT('Ctrl Pts',(29.481561161048,-7.04232459329972,-0.0439899824717745));
#31934=CARTESIAN_POINT('Ctrl Pts',(28.9652970371703,-7.37504694162997,-0.389236972868619));
#31935=CARTESIAN_POINT('Ctrl Pts',(28.9689298214357,-7.37227200661717,-0.209763874461039));
#31936=CARTESIAN_POINT('Ctrl Pts',(29.0084787340067,-7.42047716376697,-0.0414223856508554));
#31937=CARTESIAN_POINT('Ctrl Pts',(28.2150317307457,-7.8729956694109,-0.361993861939527));
#31938=CARTESIAN_POINT('Ctrl Pts',(28.2191095777036,-7.87047110758279,-0.195122273103594));
#31939=CARTESIAN_POINT('Ctrl Pts',(28.2510459088753,-7.91449073927164,-0.037280815250846));
#31940=CARTESIAN_POINT('Ctrl Pts',(27.956570399131,-8.02704348376974,-0.352282263845473));
#31941=CARTESIAN_POINT('Ctrl Pts',(27.9608114812428,-8.02460729347139,-0.189901771615212));
#31942=CARTESIAN_POINT('Ctrl Pts',(27.9899390476894,-8.06714077884413,-0.0358480736072952));
#31943=CARTESIAN_POINT('Ctrl Pts',(27.422538725282,-8.31073680629816,-0.331227233487651));
#31944=CARTESIAN_POINT('Ctrl Pts',(27.4270826096138,-8.30850613456263,-0.178579183139945));
#31945=CARTESIAN_POINT('Ctrl Pts',(27.4509872039948,-8.34755545461492,-0.0328670883961612));
#31946=CARTESIAN_POINT('Ctrl Pts',(27.1459961653714,-8.44062057060663,-0.319840425202939));
#31947=CARTESIAN_POINT('Ctrl Pts',(27.15068459432,-8.43851047177455,-0.172453929810078));
#31948=CARTESIAN_POINT('Ctrl Pts',(27.1720884374499,-8.47550022999066,-0.0313130112254784));
#31949=CARTESIAN_POINT('Ctrl Pts',(26.3082189750106,-8.78499234568452,-0.28314310589906));
#31950=CARTESIAN_POINT('Ctrl Pts',(26.3133627198456,-8.7832436968066,-0.152707180606665));
#31951=CARTESIAN_POINT('Ctrl Pts',(26.3268414702778,-8.81402640047916,-0.0265301127609303));
#31952=CARTESIAN_POINT('Ctrl Pts',(25.7337629486952,-8.95777986606701,-0.255738121841735));
#31953=CARTESIAN_POINT('Ctrl Pts',(25.7391198628699,-8.95635681278008,-0.137952410902559));
#31954=CARTESIAN_POINT('Ctrl Pts',(25.7488742137392,-8.98148038394029,-0.0232071389870805));
#31955=CARTESIAN_POINT('Ctrl Pts',(24.8488322354996,-9.13271117527261,-0.201422710338595));
#31956=CARTESIAN_POINT('Ctrl Pts',(24.85431631276,-9.13180909992311,-0.108676967321741));
#31957=CARTESIAN_POINT('Ctrl Pts',(24.8618592937854,-9.14780634343858,-0.0174743900899742));
#31958=CARTESIAN_POINT('Ctrl Pts',(24.5493473176432,-9.17693685209723,-0.181278555574678));
#31959=CARTESIAN_POINT('Ctrl Pts',(24.5548852729846,-9.17621341858475,-0.0978176119286749));
#31960=CARTESIAN_POINT('Ctrl Pts',(24.5614827959266,-9.18906214293745,-0.0154452600370327));
#31961=CARTESIAN_POINT('Ctrl Pts',(24.0962646566309,-9.22109619601667,-0.141898246278996));
#31962=CARTESIAN_POINT('Ctrl Pts',(24.1018342618134,-9.22064518679162,-0.0765766260304406));
#31963=CARTESIAN_POINT('Ctrl Pts',(24.1078835619629,-9.22867390569795,-0.0117975702348942));
#31964=CARTESIAN_POINT('Ctrl Pts',(23.9451103869883,-9.23207461097023,-0.127435185337285));
#31965=CARTESIAN_POINT('Ctrl Pts',(23.9506929727475,-9.23171479242211,-0.0687748081469021));
#31966=CARTESIAN_POINT('Ctrl Pts',(23.9565156706971,-9.23812508071924,-0.0104948818754195));
#31967=CARTESIAN_POINT('Ctrl Pts',(23.7185889926574,-9.24296254743562,-0.0993609997538649));
#31968=CARTESIAN_POINT('Ctrl Pts',(23.7241791415465,-9.24273959271718,-0.0536265938788905));
#31969=CARTESIAN_POINT('Ctrl Pts',(23.7298736629463,-9.24671619801047,-0.00808004655455183));
#31970=CARTESIAN_POINT('Ctrl Pts',(23.6430586656737,-9.2456625586093,-0.089045290078164));
#31971=CARTESIAN_POINT('Ctrl Pts',(23.6486519255516,-9.24548527128067,-0.0480602081809084));
#31972=CARTESIAN_POINT('Ctrl Pts',(23.6542931292373,-9.24864855291419,-0.00720601563352635));
#31973=CARTESIAN_POINT('Ctrl Pts',(23.5302452018234,-9.24832020150248,-0.0689516266792481));
#31974=CARTESIAN_POINT('Ctrl Pts',(23.5358401824189,-9.24821115604552,-0.0372161319416783));
#31975=CARTESIAN_POINT('Ctrl Pts',(23.5414539113024,-9.25015795747161,-0.00554437323078288));
#31976=CARTESIAN_POINT('Ctrl Pts',(23.4927698292594,-9.24897232310166,-0.0615775233974875));
#31977=CARTESIAN_POINT('Ctrl Pts',(23.4983655159144,-9.24888594108447,-0.0332364108970037));
#31978=CARTESIAN_POINT('Ctrl Pts',(23.5039677092379,-9.25042838173558,-0.00493933046707393));
#31979=CARTESIAN_POINT('Ctrl Pts',(23.437207464985,-9.24960744693864,-0.047173048025456));
#31980=CARTESIAN_POINT('Ctrl Pts',(23.4428035048708,-9.24955468884453,-0.025461954196264));
#31981=CARTESIAN_POINT('Ctrl Pts',(23.4484009772938,-9.25049704610979,-0.00377193262624975));
#31982=CARTESIAN_POINT('Ctrl Pts',(23.4187809144,-9.2497619746319,-0.0418867767987868));
#31983=CARTESIAN_POINT('Ctrl Pts',(23.4243771019783,-9.24972035740697,-0.022608789399977));
#31984=CARTESIAN_POINT('Ctrl Pts',(23.4299724616912,-9.25046369517988,-0.00334517687545925));
#31985=CARTESIAN_POINT('Ctrl Pts',(23.391639961472,-9.24991070032528,-0.0314080342235584));
#31986=CARTESIAN_POINT('Ctrl Pts',(23.3972362039634,-9.24988551015033,-0.0169528988061137));
#31987=CARTESIAN_POINT('Ctrl Pts',(23.4028313580097,-9.250335588764,-0.00250444453845097));
#31988=CARTESIAN_POINT('Ctrl Pts',(23.3826392408352,-9.24994623900697,-0.0275171890118582));
#31989=CARTESIAN_POINT('Ctrl Pts',(23.3882355060456,-9.24992647330526,-0.0148528068526551));
#31990=CARTESIAN_POINT('Ctrl Pts',(23.3938305105107,-9.25027946927614,-0.00219288882915726));
#31991=CARTESIAN_POINT('Ctrl Pts',(23.3658173417907,-9.2499903003333,-0.0174297620612975));
#31992=CARTESIAN_POINT('Ctrl Pts',(23.3714136289275,-9.24998074934077,-0.00940802009743088));
#31993=CARTESIAN_POINT('Ctrl Pts',(23.377008722703,-9.25015155434988,-0.00138747258816392));
#31994=CARTESIAN_POINT('Ctrl Pts',(23.3554916517933,-9.2499983698261,-0.011326547126086));
#31995=CARTESIAN_POINT('Ctrl Pts',(23.3610879101787,-9.24999839768389,-0.00611426124958945));
#31996=CARTESIAN_POINT('Ctrl Pts',(23.3666837799662,-9.24999842553965,-0.000902536247986865));
#31997=CARTESIAN_POINT('Ctrl Pts',(23.3560798278474,-9.24999837277875,2.22339565558631E-11));
#31998=CARTESIAN_POINT('Ctrl Pts',(23.3560798278474,-9.24999837277876,2.22339565558632E-11));
#31999=CARTESIAN_POINT('Ctrl Pts',(23.3560798278469,-9.24999837277874,2.22339565558627E-11));
#38612=UNCERTAINTY_MEASURE_WITH_UNIT(LENGTH_MEASURE(0.01),#38636,
'DISTANCE_ACCURACY_VALUE',
'Maximum model space distance between geometric entities at asserted c
onnectivities');
#38619=UNCERTAINTY_MEASURE_WITH_UNIT(LENGTH_MEASURE(0.01),#38636,
'DISTANCE_ACCURACY_VALUE',
'Maximum model space distance between geometric entities at asserted c
onnectivities');
#38628=(
GEOMETRIC_REPRESENTATION_CONTEXT(3)
GLOBAL_UNCERTAINTY_ASSIGNED_CONTEXT((#38612))
GLOBAL_UNIT_ASSIGNED_CONTEXT((#38636,#38638,#38639))
REPRESENTATION_CONTEXT('','3D')
);
#38635=(
GEOMETRIC_REPRESENTATION_CONTEXT(3)
GLOBAL_UNCERTAINTY_ASSIGNED_CONTEXT((#38619))
GLOBAL_UNIT_ASSIGNED_CONTEXT((#38636,#38638,#38639))
REPRESENTATION_CONTEXT('','3D')
);
#38636=(
LENGTH_UNIT()
NAMED_UNIT(*)
SI_UNIT(.MILLI.,.METRE.)
);
#38638=(
NAMED_UNIT(*)
PLANE_ANGLE_UNIT()
SI_UNIT($,.RADIAN.)
);
#38639=(
NAMED_UNIT(*)
SI_UNIT($,.STERADIAN.)
SOLID_ANGLE_UNIT()
);
#38648=SHAPE_DEFINITION_REPRESENTATION(#38663,#38692);
#38663=PRODUCT_DEFINITION_SHAPE('',$,#38708);
#38692=SHAPE_REPRESENTATION('',(#18058),#38628);
#38699=PRODUCT_DEFINITION_CONTEXT('part definition',#38746,'design');
#38708=PRODUCT_DEFINITION('Arm Joint 1','Arm Joint 1',#38723,#38699);
#38723=PRODUCT_DEFINITION_FORMATION('',$,#38756);
#38746=APPLICATION_CONTEXT(
'Core Data for Automotive Mechanical Design Process');
#38747=PRODUCT_CONTEXT('part definition',#38746,'mechanical');
#38756=PRODUCT('Arm Joint 1','Arm Joint 1',$,(#38747));
#38767=PRESENTATION_STYLE_ASSIGNMENT((#38774));
#38774=SURFACE_STYLE_USAGE(.BOTH.,#38781);
#38781=SURFACE_SIDE_STYLE('',(#38788));
#38788=SURFACE_STYLE_FILL_AREA(#38795);
#38795=FILL_AREA_STYLE('Opaque(97,158,199)',(#38802));
#38802=FILL_AREA_STYLE_COLOUR('Opaque(97,158,199)',#38809);
#38809=COLOUR_RGB('Opaque(97,158,199)',0.380392156862745,0.619607843137255,
0.780392156862745);
ENDSEC;
END-ISO-10303-21;
